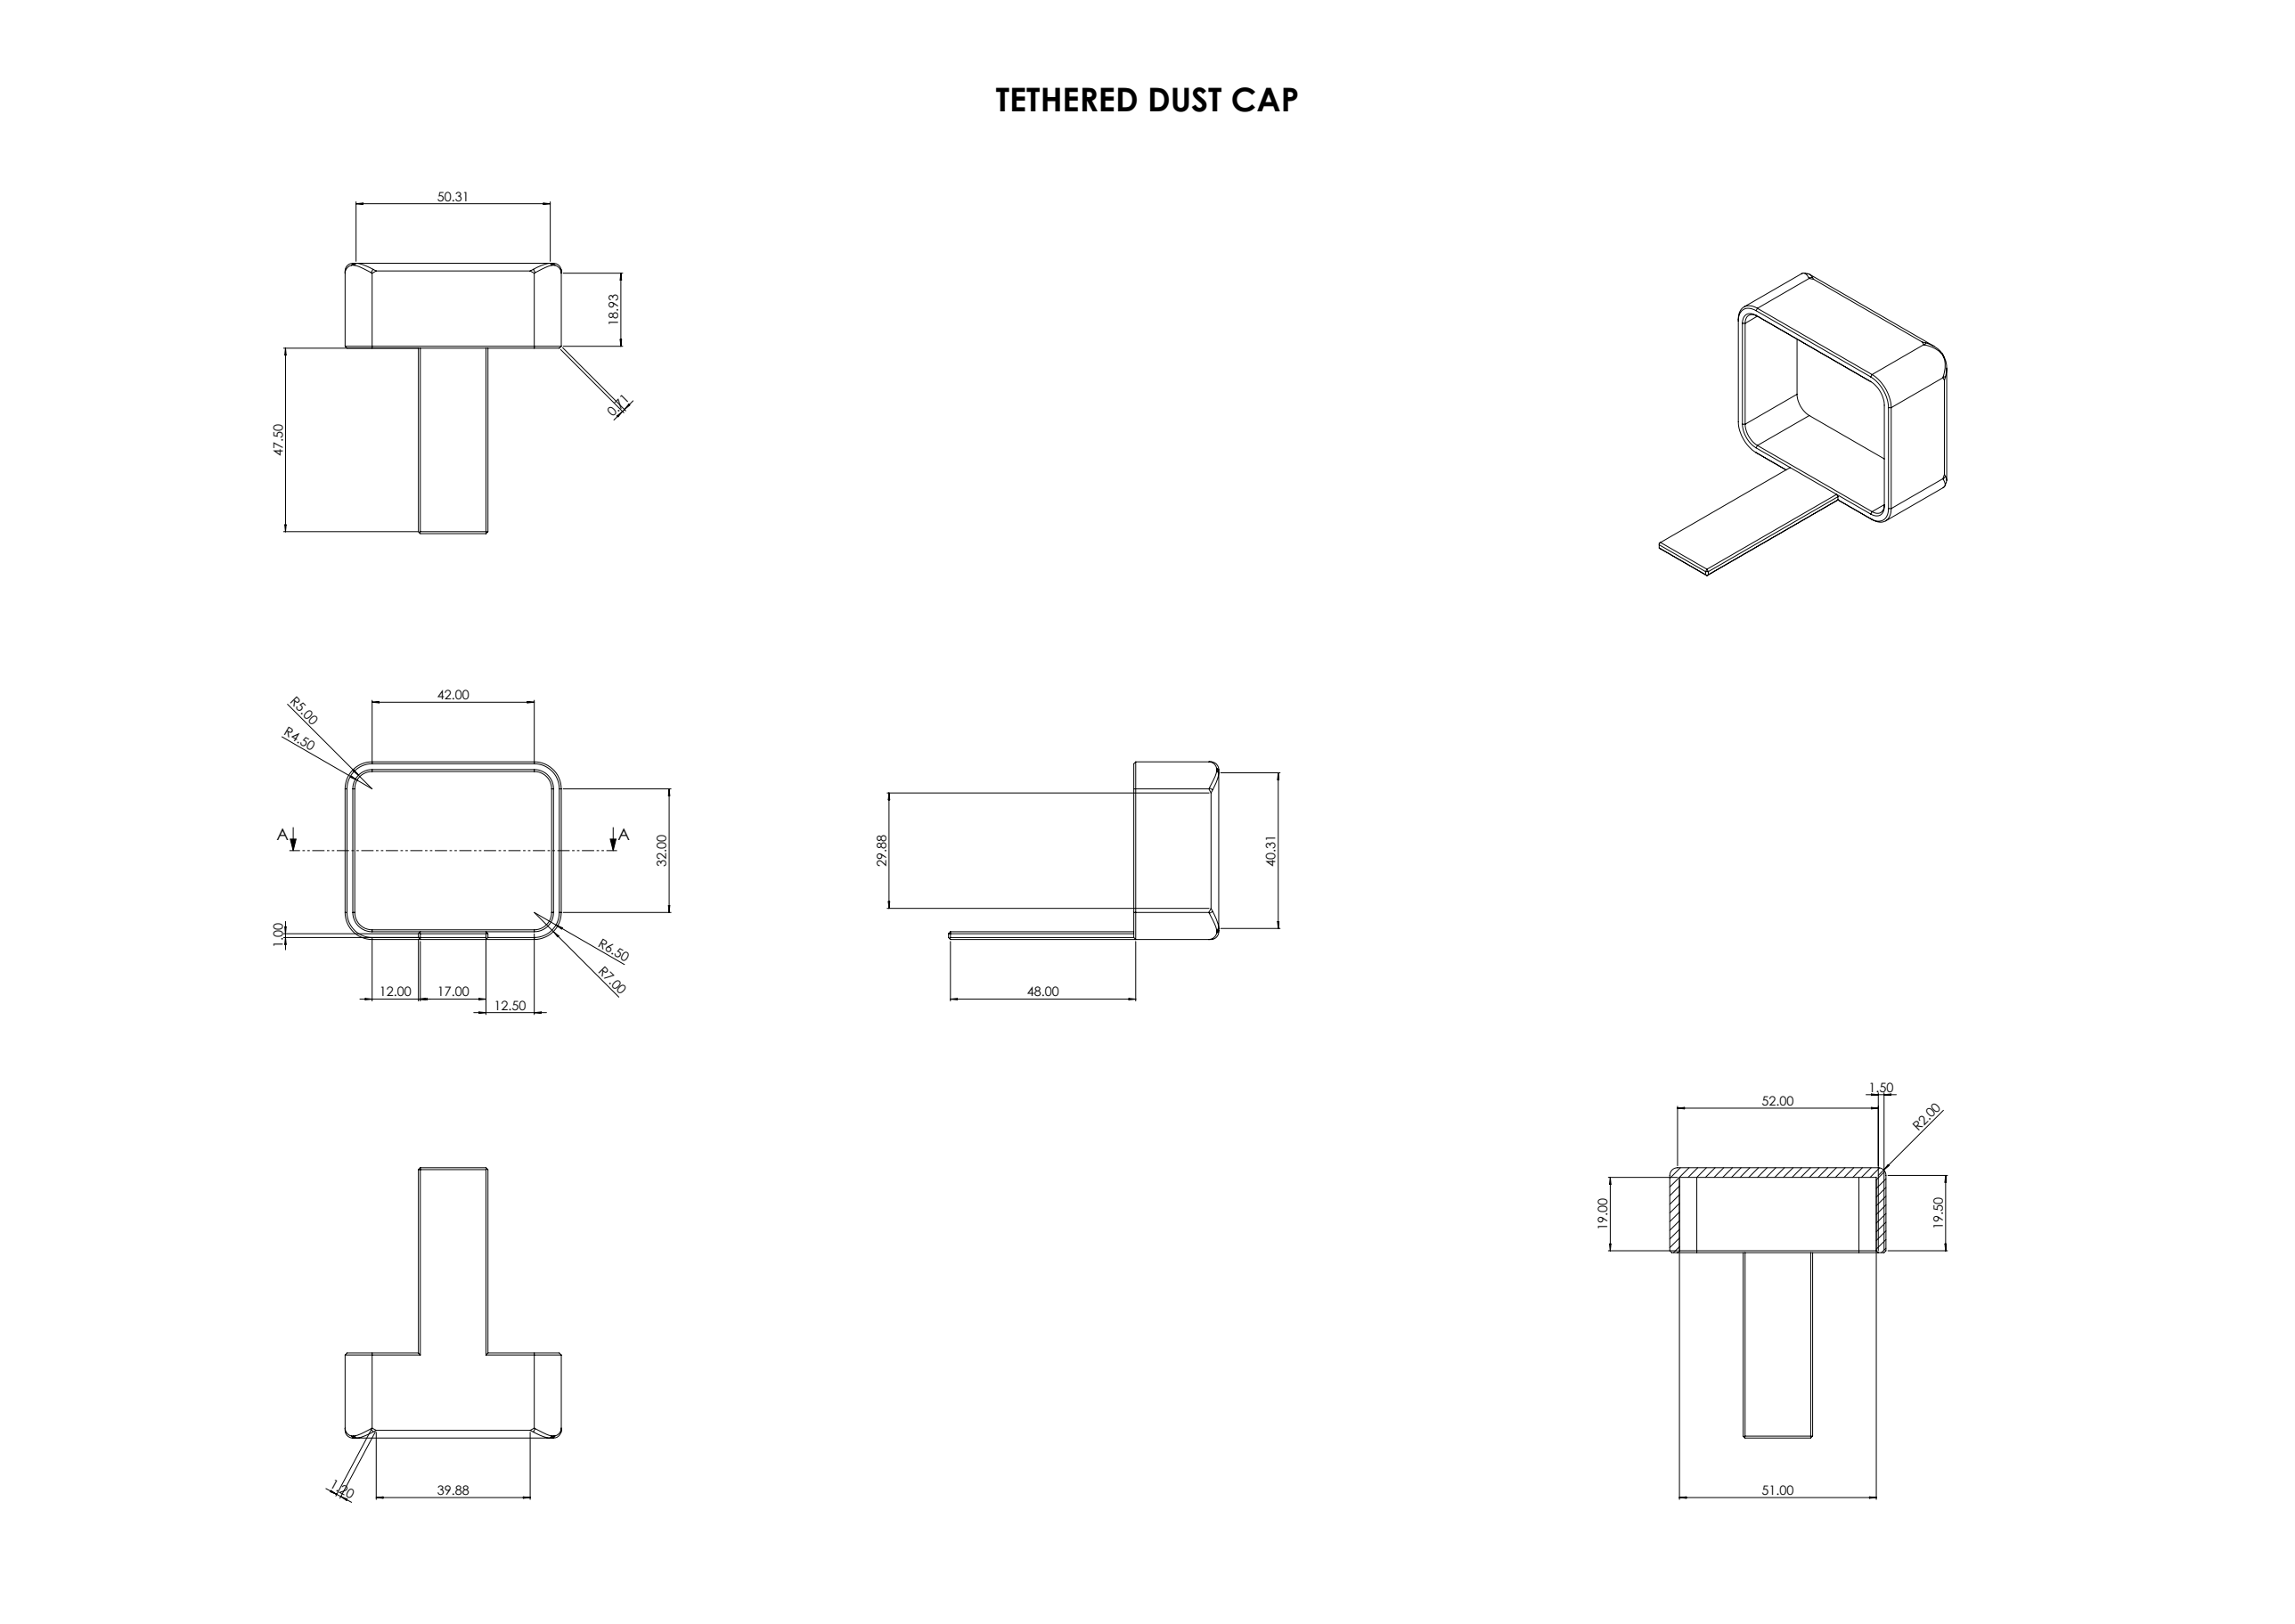
ISO-10303-21;
HEADER;
/* Generated by software containing ST-Developer
 * from STEP Tools, Inc. (www.steptools.com) 
 */

FILE_DESCRIPTION(
/* description */ (''),
/* implementation_level */ '2;1');

FILE_NAME(
/* name */ '14_Tethered_Dust_Cap.step',
/* time_stamp */ '2026-10-25T01:30:15-07:00',
/* author */ (''),
/* organization */ (''),
/* preprocessor_version */ 'ST-DEVELOPER v20.2',
/* originating_system */ 'Autodesk Translation Framework v15.15.0.0',
/* authorisation */ '');

FILE_SCHEMA (('AUTOMOTIVE_DESIGN { 1 0 10303 214 3 1 1 }'));
ENDSEC;

DATA;
#10=MECHANICAL_DESIGN_GEOMETRIC_PRESENTATION_REPRESENTATION('',(#575),#32309);
#87=(
BOUNDED_CURVE()
B_SPLINE_CURVE(3,(#30768,#30769,#30770,#30771,#30772,#30773,#30774,#30775,
#30776,#30777,#30778,#30779),.UNSPECIFIED.,.F.,.F.)
B_SPLINE_CURVE_WITH_KNOTS((4,2,2,2,2,4),(0.000100085581199306,0.11804875878528,
0.236101413685198,0.384034650166034,0.497829447458985,0.511841573844537),
 .UNSPECIFIED.)
CURVE()
GEOMETRIC_REPRESENTATION_ITEM()
RATIONAL_B_SPLINE_CURVE((1.,1.,1.,1.,1.,1.,1.,1.,1.,1.,1.,1.))
REPRESENTATION_ITEM('')
);
#352=B_SPLINE_CURVE_WITH_KNOTS('',3,(#29537,#29538,#29539,#29540,#29541,
#29542,#29543,#29544,#29545,#29546,#29547,#29548,#29549,#29550,#29551,#29552,
#29553,#29554,#29555,#29556,#29557,#29558,#29559,#29560,#29561,#29562,#29563,
#29564,#29565,#29566,#29567,#29568,#29569,#29570,#29571,#29572,#29573,#29574,
#29575,#29576,#29577,#29578,#29579,#29580,#29581,#29582,#29583,#29584,#29585,
#29586,#29587,#29588,#29589,#29590,#29591,#29592,#29593,#29594,#29595,#29596,
#29597,#29598,#29599,#29600,#29601,#29602,#29603,#29604,#29605,#29606,#29607,
#29608,#29609,#29610,#29611,#29612,#29613,#29614,#29615,#29616,#29617,#29618,
#29619,#29620,#29621,#29622,#29623,#29624,#29625,#29626,#29627,#29628,#29629,
#29630),.UNSPECIFIED.,.F.,.F.,(4,3,3,3,3,3,3,3,3,3,3,3,3,3,3,3,3,3,3,3,
3,3,3,3,3,3,3,3,3,3,3,4),(0.,0.0258707374451698,0.0523995842804884,0.0797001065242145,
0.108495122701971,0.138579548146388,0.170391094738405,0.204740918376836,
0.243564930469247,0.301738535677522,0.342786820776585,0.377562328700043,
0.409462754742929,0.439523776912731,0.468248829463879,0.497342034867759,
0.525270549115699,0.554941139795967,0.585586421921526,0.618112000252219,
0.653483627180876,0.694829905002005,0.747358415243329,0.784774064435163,
0.818382572828511,0.849773402002612,0.879622020764925,0.909716515573693,
0.937043932385008,0.963754510580494,0.989696242215803,1.),.UNSPECIFIED.);
#353=B_SPLINE_CURVE_WITH_KNOTS('',3,(#29632,#29633,#29634,#29635),
 .UNSPECIFIED.,.F.,.F.,(4,4),(-1.,0.),.UNSPECIFIED.);
#354=B_SPLINE_CURVE_WITH_KNOTS('',3,(#29637,#29638,#29639,#29640,#29641,
#29642,#29643,#29644,#29645,#29646,#29647,#29648,#29649,#29650,#29651,#29652,
#29653,#29654,#29655,#29656,#29657,#29658,#29659,#29660,#29661,#29662,#29663,
#29664,#29665,#29666,#29667,#29668,#29669,#29670,#29671,#29672,#29673,#29674,
#29675,#29676,#29677,#29678,#29679,#29680,#29681,#29682,#29683,#29684,#29685,
#29686,#29687,#29688,#29689,#29690,#29691,#29692,#29693,#29694,#29695,#29696,
#29697,#29698,#29699,#29700,#29701,#29702,#29703,#29704,#29705,#29706),
 .UNSPECIFIED.,.F.,.F.,(4,3,3,3,3,3,3,3,3,3,3,3,3,3,3,3,3,3,3,3,3,3,3,4),
(0.,0.0359057501184,0.0731782994099124,0.112196676257152,0.153588188584124,
0.19856311186321,0.251379995782812,0.322351118570897,0.369695903527712,
0.412227930465316,0.451958538122157,0.49032799292638,0.52995524039796,0.570194128050318,
0.613255077113093,0.66118815818441,0.72826108783719,0.783703920872222,0.829758018851651,
0.872318514138739,0.910997179683127,0.94830001070203,0.984014129742057,
1.),.UNSPECIFIED.);
#355=B_SPLINE_CURVE_WITH_KNOTS('',3,(#29742,#29743,#29744,#29745,#29746,
#29747,#29748,#29749,#29750,#29751,#29752,#29753,#29754,#29755,#29756,#29757,
#29758,#29759,#29760,#29761,#29762,#29763,#29764,#29765,#29766,#29767,#29768,
#29769,#29770,#29771,#29772,#29773,#29774,#29775,#29776,#29777,#29778,#29779,
#29780,#29781,#29782,#29783,#29784,#29785,#29786,#29787,#29788,#29789,#29790,
#29791,#29792,#29793,#29794,#29795,#29796,#29797,#29798,#29799,#29800,#29801,
#29802,#29803,#29804,#29805,#29806,#29807,#29808,#29809,#29810,#29811),
 .UNSPECIFIED.,.F.,.F.,(4,3,3,3,3,3,3,3,3,3,3,3,3,3,3,3,3,3,3,3,3,3,3,4),
(0.,0.0359049134463849,0.073176547549646,0.112193893168169,0.153584182812285,
0.198557501853783,0.251370838267118,0.322351741442161,0.369695708180622,
0.412227003870618,0.451956929703973,0.490325803323821,0.529954284988624,
0.570193684366073,0.613255163900098,0.661188823039329,0.728261735081395,
0.783705956052361,0.829760865743545,0.872320649307659,0.91099999721276,
0.948303461797003,0.984018202039666,1.),.UNSPECIFIED.);
#356=B_SPLINE_CURVE_WITH_KNOTS('',3,(#29813,#29814,#29815,#29816),
 .UNSPECIFIED.,.F.,.F.,(4,4),(0.,1.),.UNSPECIFIED.);
#357=B_SPLINE_CURVE_WITH_KNOTS('',3,(#29818,#29819,#29820,#29821,#29822,
#29823,#29824,#29825,#29826,#29827,#29828,#29829,#29830,#29831,#29832,#29833,
#29834,#29835,#29836,#29837,#29838,#29839,#29840,#29841,#29842,#29843,#29844,
#29845,#29846,#29847,#29848,#29849,#29850,#29851,#29852,#29853,#29854,#29855,
#29856,#29857,#29858,#29859,#29860,#29861,#29862,#29863,#29864,#29865,#29866,
#29867,#29868,#29869,#29870,#29871,#29872,#29873,#29874,#29875,#29876,#29877,
#29878,#29879,#29880,#29881,#29882,#29883,#29884,#29885,#29886,#29887,#29888,
#29889,#29890,#29891,#29892,#29893,#29894,#29895,#29896,#29897,#29898,#29899,
#29900,#29901,#29902,#29903,#29904,#29905,#29906,#29907,#29908,#29909,#29910,
#29911),.UNSPECIFIED.,.F.,.F.,(4,3,3,3,3,3,3,3,3,3,3,3,3,3,3,3,3,3,3,3,
3,3,3,3,3,3,3,3,3,3,3,4),(0.,0.0258806755131893,0.0524200922167716,0.0797320051430074,
0.108539985769749,0.138639209785132,0.170468542508365,0.204841962640731,
0.243705620941324,0.301747786726151,0.342801252332619,0.377583664170473,
0.409491204995713,0.439559328397146,0.468291405426299,0.497246492955408,
0.525185050106943,0.554860984475259,0.585493446299901,0.618003829089383,
0.653355383451557,0.694654043666211,0.747235195717053,0.784647728535492,
0.818250751836891,0.849635399921593,0.879477588119271,0.909608191089453,
0.936927404966159,0.963630037681853,0.989563296559285,1.),.UNSPECIFIED.);
#358=B_SPLINE_CURVE_WITH_KNOTS('',3,(#29934,#29935,#29936,#29937,#29938),
 .UNSPECIFIED.,.F.,.F.,(4,1,4),(0.000100085581199305,0.2925237931603,0.511841573844625),
 .UNSPECIFIED.);
#359=B_SPLINE_CURVE_WITH_KNOTS('',3,(#29941,#29942,#29943,#29944,#29945),
 .UNSPECIFIED.,.F.,.F.,(4,1,4),(-0.511841573844625,-0.2925237931603,-0.000100085581199305),
 .UNSPECIFIED.);
#360=B_SPLINE_CURVE_WITH_KNOTS('',3,(#29971,#29972,#29973,#29974),
 .UNSPECIFIED.,.F.,.F.,(4,4),(-0.568951195767079,-0.511841573844535),
 .UNSPECIFIED.);
#361=B_SPLINE_CURVE_WITH_KNOTS('',3,(#29975,#29976,#29977,#29978),
 .UNSPECIFIED.,.F.,.F.,(4,4),(0.511841573844535,0.568951195767079),
 .UNSPECIFIED.);
#362=B_SPLINE_CURVE_WITH_KNOTS('',3,(#30000,#30001,#30002,#30003,#30004),
 .UNSPECIFIED.,.F.,.F.,(4,1,4),(-1.80301165508774,-1.58369377785584,-1.29126994154665),
 .UNSPECIFIED.);
#363=B_SPLINE_CURVE_WITH_KNOTS('',3,(#30007,#30008,#30009,#30010,#30011),
 .UNSPECIFIED.,.F.,.F.,(4,1,4),(1.29126994154665,1.58369377785584,1.80301165508774),
 .UNSPECIFIED.);
#364=B_SPLINE_CURVE_WITH_KNOTS('',3,(#30028,#30029,#30030,#30031),
 .UNSPECIFIED.,.F.,.F.,(4,4),(-1.29126994154674,-1.2341603196242),
 .UNSPECIFIED.);
#365=B_SPLINE_CURVE_WITH_KNOTS('',3,(#30032,#30033,#30034,#30035),
 .UNSPECIFIED.,.F.,.F.,(4,4),(1.2341603196242,1.29126994154674),
 .UNSPECIFIED.);
#366=B_SPLINE_CURVE_WITH_KNOTS('',3,(#30040,#30041,#30042,#30043,#30044,
#30045,#30046,#30047,#30048,#30049,#30050,#30051,#30052,#30053,#30054,#30055,
#30056,#30057,#30058,#30059,#30060,#30061,#30062,#30063,#30064,#30065,#30066,
#30067,#30068,#30069,#30070,#30071,#30072,#30073,#30074,#30075,#30076,#30077,
#30078,#30079,#30080,#30081,#30082,#30083,#30084,#30085,#30086,#30087,#30088,
#30089,#30090,#30091,#30092,#30093,#30094,#30095,#30096,#30097,#30098,#30099,
#30100,#30101,#30102,#30103,#30104,#30105,#30106,#30107,#30108,#30109,#30110,
#30111,#30112,#30113,#30114,#30115,#30116,#30117,#30118,#30119,#30120,#30121,
#30122,#30123,#30124,#30125,#30126,#30127,#30128,#30129,#30130,#30131,#30132,
#30133),.UNSPECIFIED.,.F.,.F.,(4,3,3,3,3,3,3,3,3,3,3,3,3,3,3,3,3,3,3,3,
3,3,3,3,3,3,3,3,3,3,3,4),(0.,0.0258806755478976,0.0524200922876265,0.0797320052517776,
0.108539985919231,0.138639209979136,0.170468542753168,0.204841962945636,
0.243705621312987,0.301747784910779,0.34280125092102,0.377583662940723,
0.409491203889412,0.439559327385709,0.468291404493187,0.49724649358827,
0.525185050645796,0.554860984980434,0.585493446871105,0.61800382974593,
0.653355384235859,0.694654044834357,0.747235196465702,0.78464772923462,
0.818250752522057,0.849635400605874,0.879477588809083,0.909608191606812,
0.936927405502566,0.963630038237505,0.989563297137722,1.),.UNSPECIFIED.);
#367=B_SPLINE_CURVE_WITH_KNOTS('',3,(#30135,#30136,#30137,#30138,#30139),
 .UNSPECIFIED.,.F.,.F.,(4,1,4),(-0.511841573844626,-0.2925237931603,-0.000100085581199306),
 .UNSPECIFIED.);
#368=B_SPLINE_CURVE_WITH_KNOTS('',3,(#30195,#30196,#30197,#30198,#30199,
#30200,#30201,#30202,#30203,#30204,#30205,#30206,#30207,#30208,#30209,#30210,
#30211,#30212,#30213,#30214,#30215,#30216,#30217,#30218,#30219,#30220,#30221,
#30222,#30223,#30224,#30225,#30226,#30227,#30228,#30229,#30230,#30231,#30232,
#30233,#30234,#30235,#30236,#30237,#30238,#30239,#30240,#30241,#30242,#30243,
#30244,#30245,#30246,#30247,#30248,#30249,#30250,#30251,#30252,#30253,#30254,
#30255,#30256,#30257,#30258,#30259,#30260,#30261,#30262,#30263,#30264,#30265,
#30266,#30267,#30268,#30269,#30270,#30271,#30272,#30273,#30274,#30275,#30276,
#30277,#30278,#30279,#30280,#30281,#30282,#30283,#30284,#30285,#30286,#30287,
#30288),.UNSPECIFIED.,.F.,.F.,(4,3,3,3,3,3,3,3,3,3,3,3,3,3,3,3,3,3,3,3,
3,3,3,3,3,3,3,3,3,3,3,4),(0.,0.0258707373852982,0.0523995841574412,0.0797001063343714,
0.108495122436769,0.138579547796529,0.170391094289058,0.204740917798661,
0.243564929672972,0.301738533531649,0.342786818919582,0.377562326926431,
0.409462753002346,0.439523775182168,0.468248827730827,0.497342036568372,
0.525270550411946,0.554941141011199,0.585586423119629,0.618112001453677,
0.653483628442009,0.694829906775482,0.747358417163163,0.784774066048828,
0.818382574240286,0.849773403259427,0.87962202189283,0.909716516419622,
0.937043933139065,0.963754511246871,0.989696242803908,1.),.UNSPECIFIED.);
#369=B_SPLINE_CURVE_WITH_KNOTS('',3,(#30290,#30291,#30292,#30293),
 .UNSPECIFIED.,.F.,.F.,(4,4),(-1.,0.),.UNSPECIFIED.);
#370=B_SPLINE_CURVE_WITH_KNOTS('',3,(#30295,#30296,#30297,#30298,#30299,
#30300,#30301,#30302,#30303,#30304,#30305,#30306,#30307,#30308,#30309,#30310,
#30311,#30312,#30313,#30314,#30315,#30316,#30317,#30318,#30319,#30320,#30321,
#30322,#30323,#30324,#30325,#30326,#30327,#30328,#30329,#30330,#30331,#30332,
#30333,#30334,#30335,#30336,#30337,#30338,#30339,#30340,#30341,#30342,#30343,
#30344,#30345,#30346,#30347,#30348,#30349,#30350,#30351,#30352,#30353,#30354,
#30355,#30356,#30357,#30358,#30359,#30360,#30361,#30362,#30363,#30364),
 .UNSPECIFIED.,.F.,.F.,(4,3,3,3,3,3,3,3,3,3,3,3,3,3,3,3,3,3,3,3,3,3,3,4),
(0.,0.0359057503974645,0.0731782999903264,0.112196677171334,0.153588189884582,
0.198563113652405,0.251379998572626,0.322351119089413,0.369695904344816,
0.412227931549056,0.45195853945437,0.490327994460789,0.529955241857638,
0.570194129909524,0.613255079462038,0.661188161329761,0.728261095682754,
0.783703926991951,0.829758024663586,0.872318518497689,0.910997184172885,
0.948300015335705,0.984014134572557,1.),.UNSPECIFIED.);
#371=B_SPLINE_CURVE_WITH_KNOTS('',3,(#30399,#30400,#30401,#30402,#30403,
#30404,#30405,#30406,#30407,#30408,#30409,#30410,#30411,#30412,#30413,#30414,
#30415,#30416,#30417,#30418,#30419,#30420,#30421,#30422,#30423,#30424,#30425,
#30426,#30427,#30428,#30429,#30430,#30431,#30432,#30433,#30434,#30435,#30436,
#30437,#30438,#30439,#30440,#30441,#30442,#30443,#30444,#30445,#30446,#30447,
#30448,#30449,#30450,#30451,#30452,#30453,#30454,#30455,#30456,#30457,#30458,
#30459,#30460,#30461,#30462,#30463,#30464,#30465,#30466,#30467,#30468),
 .UNSPECIFIED.,.F.,.F.,(4,3,3,3,3,3,3,3,3,3,3,3,3,3,3,3,3,3,3,3,3,3,3,4),
(0.,0.0359049133077996,0.0731765472614101,0.112193892714089,0.153584182166311,
0.198557500964563,0.251370836880033,0.322351741174105,0.369695707765568,
0.412227003323922,0.451956929034388,0.490325802554425,0.529954284258119,
0.5701936834371,0.613255162727241,0.661188821470719,0.728261731182501,0.783705953011855,
0.829760862856234,0.872320647142176,0.910999994982448,0.948303459495199,
0.984018199640234,1.),.UNSPECIFIED.);
#372=B_SPLINE_CURVE_WITH_KNOTS('',3,(#30469,#30470,#30471,#30472),
 .UNSPECIFIED.,.F.,.F.,(4,4),(0.,1.),.UNSPECIFIED.);
#373=B_SPLINE_CURVE_WITH_KNOTS('',3,(#30494,#30495,#30496,#30497,#30498),
 .UNSPECIFIED.,.F.,.F.,(4,1,4),(0.000100085581199306,0.2925237931603,0.511841573844626),
 .UNSPECIFIED.);
#374=B_SPLINE_CURVE_WITH_KNOTS('',3,(#30525,#30526,#30527,#30528),
 .UNSPECIFIED.,.F.,.F.,(4,4),(-0.568951195767079,-0.511841573844535),
 .UNSPECIFIED.);
#375=B_SPLINE_CURVE_WITH_KNOTS('',3,(#30529,#30530,#30531,#30532),
 .UNSPECIFIED.,.F.,.F.,(4,4),(0.511841573844535,0.568951195767079),
 .UNSPECIFIED.);
#376=B_SPLINE_CURVE_WITH_KNOTS('',3,(#30554,#30555,#30556,#30557,#30558),
 .UNSPECIFIED.,.F.,.F.,(4,1,4),(-1.82014070277373,-1.52771686646454,-1.30839898923264),
 .UNSPECIFIED.);
#377=B_SPLINE_CURVE_WITH_KNOTS('',3,(#30561,#30562,#30563,#30564,#30565),
 .UNSPECIFIED.,.F.,.F.,(4,1,4),(1.30839898923264,1.52771686646454,1.82014070277373),
 .UNSPECIFIED.);
#378=B_SPLINE_CURVE_WITH_KNOTS('',3,(#30582,#30583,#30584,#30585),
 .UNSPECIFIED.,.F.,.F.,(4,4),(-1.30839898923273,-1.25128936731019),
 .UNSPECIFIED.);
#379=B_SPLINE_CURVE_WITH_KNOTS('',3,(#30586,#30587,#30588,#30589),
 .UNSPECIFIED.,.F.,.F.,(4,4),(1.25128936731019,1.30839898923273),
 .UNSPECIFIED.);
#380=B_SPLINE_CURVE_WITH_KNOTS('',3,(#30594,#30595,#30596,#30597),
 .UNSPECIFIED.,.F.,.F.,(4,4),(-0.568951195767077,-0.511841573844537),
 .UNSPECIFIED.);
#381=B_SPLINE_CURVE_WITH_KNOTS('',3,(#30601,#30602,#30603,#30604),
 .UNSPECIFIED.,.F.,.F.,(4,4),(-1.30839898923273,-1.25128936731019),
 .UNSPECIFIED.);
#382=B_SPLINE_CURVE_WITH_KNOTS('',3,(#30608,#30609,#30610,#30611),
 .UNSPECIFIED.,.F.,.F.,(4,4),(-0.568951195767079,-0.511841573844536),
 .UNSPECIFIED.);
#383=B_SPLINE_CURVE_WITH_KNOTS('',3,(#30615,#30616,#30617,#30618),
 .UNSPECIFIED.,.F.,.F.,(4,4),(-1.29126994154674,-1.2341603196242),
 .UNSPECIFIED.);
#384=B_SPLINE_CURVE_WITH_KNOTS('',3,(#30679,#30680,#30681,#30682,#30683,
#30684,#30685,#30686,#30687,#30688,#30689,#30690,#30691,#30692,#30693,#30694,
#30695,#30696,#30697,#30698,#30699,#30700,#30701,#30702,#30703,#30704,#30705,
#30706,#30707,#30708,#30709,#30710,#30711,#30712,#30713,#30714,#30715,#30716,
#30717,#30718,#30719,#30720,#30721,#30722,#30723,#30724,#30725,#30726,#30727,
#30728,#30729,#30730,#30731,#30732,#30733,#30734,#30735,#30736,#30737,#30738,
#30739,#30740,#30741,#30742,#30743,#30744,#30745,#30746,#30747,#30748),
 .UNSPECIFIED.,.F.,.F.,(4,3,3,3,3,3,3,3,3,3,3,3,3,3,3,3,3,3,3,3,3,3,3,4),
(0.,0.0359057503975373,0.0731782999904773,0.112196677171571,0.153588189884912,
0.198563113652762,0.251379998573341,0.322351119089333,0.36969590434482,
0.412227931549108,0.451958539454481,0.490327994460949,0.529955241857821,
0.570194129909769,0.613255079462367,0.66118816133035,0.728261095684453,
0.783703926993341,0.829758024664918,0.872318518498689,0.910997184173894,
0.948300015336798,0.98401413457368,1.),.UNSPECIFIED.);
#385=B_SPLINE_CURVE_WITH_KNOTS('',3,(#30750,#30751,#30752,#30753,#30754),
 .UNSPECIFIED.,.F.,.F.,(4,1,4),(1.30839898923264,1.52771686646453,1.82014070277373),
 .UNSPECIFIED.);
#386=B_SPLINE_CURVE_WITH_KNOTS('',3,(#30756,#30757,#30758,#30759),
 .UNSPECIFIED.,.F.,.F.,(4,4),(1.25128936731019,1.30839898923273),
 .UNSPECIFIED.);
#387=B_SPLINE_CURVE_WITH_KNOTS('',3,(#30763,#30764,#30765,#30766),
 .UNSPECIFIED.,.F.,.F.,(4,4),(0.511841573844537,0.568951195767077),
 .UNSPECIFIED.);
#388=B_SPLINE_CURVE_WITH_KNOTS('',3,(#30780,#30781,#30782,#30783,#30784,
#30785,#30786,#30787,#30788,#30789,#30790,#30791,#30792,#30793,#30794,#30795,
#30796,#30797,#30798,#30799,#30800,#30801,#30802,#30803,#30804,#30805,#30806,
#30807,#30808,#30809,#30810,#30811,#30812,#30813,#30814,#30815,#30816,#30817,
#30818,#30819,#30820,#30821,#30822,#30823,#30824,#30825,#30826,#30827,#30828,
#30829,#30830,#30831,#30832,#30833,#30834,#30835,#30836,#30837,#30838,#30839,
#30840,#30841,#30842,#30843,#30844,#30845,#30846,#30847,#30848,#30849),
 .UNSPECIFIED.,.F.,.F.,(4,3,3,3,3,3,3,3,3,3,3,3,3,3,3,3,3,3,3,3,3,3,3,4),
(0.,0.0359049130301229,0.073176546683956,0.112193891804418,0.153584180872903,
0.198557499184731,0.251370834104054,0.322351740640927,0.369695706937292,
0.412227002231532,0.451956927695583,0.490325801015499,0.529954282797085,
0.570193681578136,0.613255160380649,0.661188818329747,0.72826172337588,
0.783705946924147,0.829760857074988,0.872320642806241,0.910999990516432,
0.948303454885518,0.984018194834891,1.),.UNSPECIFIED.);
#389=B_SPLINE_CURVE_WITH_KNOTS('',3,(#30894,#30895,#30896,#30897,#30898,
#30899,#30900,#30901,#30902,#30903,#30904,#30905,#30906,#30907,#30908,#30909,
#30910,#30911,#30912,#30913,#30914,#30915,#30916,#30917,#30918,#30919,#30920,
#30921,#30922,#30923,#30924,#30925,#30926,#30927,#30928,#30929,#30930,#30931,
#30932,#30933,#30934,#30935,#30936,#30937,#30938,#30939,#30940,#30941,#30942,
#30943,#30944,#30945,#30946,#30947,#30948,#30949,#30950,#30951,#30952,#30953,
#30954,#30955,#30956,#30957,#30958,#30959,#30960,#30961,#30962,#30963,#30964,
#30965,#30966,#30967,#30968,#30969,#30970,#30971,#30972,#30973,#30974,#30975,
#30976,#30977,#30978,#30979,#30980,#30981,#30982,#30983,#30984,#30985,#30986,
#30987),.UNSPECIFIED.,.F.,.F.,(4,3,3,3,3,3,3,3,3,3,3,3,3,3,3,3,3,3,3,3,
3,3,3,3,3,3,3,3,3,3,3,4),(0.,0.0258707373554823,0.0523995840965019,0.0797001062399438,
0.108495122304716,0.13857954762218,0.170391094064582,0.204740917510112,
0.243564929276073,0.301738532460215,0.342786817991936,0.377562326039311,
0.409462752131609,0.4395237743171,0.468248826864701,0.497342037419088,0.525270551060381,
0.554941141619107,0.585586423719045,0.618112002054742,0.653483629073077,
0.694829907664093,0.747358418123701,0.784774066856292,0.818382574947157,
0.849773403889227,0.879622022458522,0.909716516843892,0.937043933517235,
0.963754511581492,0.989696243099283,1.),.UNSPECIFIED.);
#390=B_SPLINE_CURVE_WITH_KNOTS('',3,(#30989,#30990,#30991,#30992),
 .UNSPECIFIED.,.F.,.F.,(4,4),(-1.,0.),.UNSPECIFIED.);
#391=B_SPLINE_CURVE_WITH_KNOTS('',3,(#30994,#30995,#30996,#30997,#30998,
#30999,#31000,#31001,#31002,#31003,#31004,#31005,#31006,#31007,#31008,#31009,
#31010,#31011,#31012,#31013,#31014,#31015,#31016,#31017,#31018,#31019,#31020,
#31021,#31022,#31023,#31024,#31025,#31026,#31027,#31028,#31029,#31030,#31031,
#31032,#31033,#31034,#31035,#31036,#31037,#31038,#31039,#31040,#31041,#31042,
#31043,#31044,#31045,#31046,#31047,#31048,#31049,#31050,#31051,#31052,#31053,
#31054,#31055,#31056,#31057,#31058,#31059,#31060,#31061,#31062,#31063),
 .UNSPECIFIED.,.F.,.F.,(4,3,3,3,3,3,3,3,3,3,3,3,3,3,3,3,3,3,3,3,3,3,3,4),
(0.,0.0359057505369141,0.0731783002803435,0.112196677628097,0.153588190534333,
0.19856311454628,0.251379999966526,0.322351119348276,0.369695904752862,
0.412227932090299,0.451958540119749,0.490327995227232,0.529955242586758,
0.570194130838204,0.613255080635413,0.66118816290105,0.728261099602057,
0.783703930049219,0.829758027567063,0.872318520675297,0.910997186415849,
0.948300017650692,0.984014136985868,1.),.UNSPECIFIED.);
#392=B_SPLINE_CURVE_WITH_KNOTS('',3,(#31099,#31100,#31101,#31102,#31103,
#31104,#31105,#31106,#31107,#31108,#31109,#31110,#31111,#31112,#31113,#31114,
#31115,#31116,#31117,#31118,#31119,#31120,#31121,#31122,#31123,#31124,#31125,
#31126,#31127,#31128,#31129,#31130,#31131,#31132,#31133,#31134,#31135,#31136,
#31137,#31138,#31139,#31140,#31141,#31142,#31143,#31144,#31145,#31146,#31147,
#31148,#31149,#31150,#31151,#31152,#31153,#31154,#31155,#31156,#31157,#31158,
#31159,#31160,#31161,#31162,#31163,#31164,#31165,#31166,#31167,#31168),
 .UNSPECIFIED.,.F.,.F.,(4,3,3,3,3,3,3,3,3,3,3,3,3,3,3,3,3,3,3,3,3,3,3,4),
(0.,0.0359049130299729,0.0731765466835763,0.112193891804017,0.153584180872098,
0.198557499183881,0.251370834102748,0.322351740640327,0.369695706936552,
0.41222700223062,0.451956927694618,0.490325801013735,0.529954282795424,
0.570193681576247,0.613255160378796,0.661188818327897,0.728261723370456,
0.783705946920119,0.829760857071578,0.872320642803683,0.910999990513864,
0.948303454883392,0.984018194832596,1.),.UNSPECIFIED.);
#393=B_SPLINE_CURVE_WITH_KNOTS('',3,(#31170,#31171,#31172,#31173),
 .UNSPECIFIED.,.F.,.F.,(4,4),(0.,1.),.UNSPECIFIED.);
#394=B_SPLINE_CURVE_WITH_KNOTS('',3,(#31175,#31176,#31177,#31178,#31179,
#31180,#31181,#31182,#31183,#31184,#31185,#31186,#31187,#31188,#31189,#31190,
#31191,#31192,#31193,#31194,#31195,#31196,#31197,#31198,#31199,#31200,#31201,
#31202,#31203,#31204,#31205,#31206,#31207,#31208,#31209,#31210,#31211,#31212,
#31213,#31214,#31215,#31216,#31217,#31218,#31219,#31220,#31221,#31222,#31223,
#31224,#31225,#31226,#31227,#31228,#31229,#31230,#31231,#31232,#31233,#31234,
#31235,#31236,#31237,#31238,#31239,#31240,#31241,#31242,#31243,#31244,#31245,
#31246,#31247,#31248,#31249,#31250,#31251,#31252,#31253,#31254,#31255,#31256,
#31257,#31258,#31259,#31260,#31261,#31262,#31263,#31264,#31265,#31266,#31267,
#31268),.UNSPECIFIED.,.F.,.F.,(4,3,3,3,3,3,3,3,3,3,3,3,3,3,3,3,3,3,3,3,
3,3,3,3,3,3,3,3,3,3,3,4),(0.,0.0258806756174258,0.052420092429605,0.0797320054697036,
0.108539986218788,0.138639210368191,0.170468543243868,0.204841963556246,
0.243705622058159,0.301747781272309,0.342801248093589,0.377583660478043,
0.409491201673175,0.439559325359787,0.468291402624354,0.497246494854993,
0.525185051724753,0.554860985991956,0.585493448014801,0.618003831060507,
0.653355385806342,0.694654047173711,0.747235197965173,0.78464773063489,
0.818250753894271,0.849635401976391,0.879477590190491,0.909608192642869,
0.936927406576889,0.963630039350146,0.989563298296144,1.),.UNSPECIFIED.);
#395=B_SPLINE_CURVE_WITH_KNOTS('',3,(#31291,#31292,#31293,#31294,#31295),
 .UNSPECIFIED.,.F.,.F.,(4,1,4),(0.000100085581199305,0.2925237931603,0.511841573844626),
 .UNSPECIFIED.);
#396=B_SPLINE_CURVE_WITH_KNOTS('',3,(#31297,#31298,#31299,#31300,#31301),
 .UNSPECIFIED.,.F.,.F.,(4,1,4),(-0.511841573844626,-0.2925237931603,-0.000100085581199305),
 .UNSPECIFIED.);
#397=B_SPLINE_CURVE_WITH_KNOTS('',3,(#31324,#31325,#31326,#31327),
 .UNSPECIFIED.,.F.,.F.,(4,4),(0.511841573844536,0.568951195767079),
 .UNSPECIFIED.);
#398=B_SPLINE_CURVE_WITH_KNOTS('',3,(#31348,#31349,#31350,#31351,#31352),
 .UNSPECIFIED.,.F.,.F.,(4,1,4),(-1.80301165508774,-1.58369377785584,-1.29126994154665),
 .UNSPECIFIED.);
#399=B_SPLINE_CURVE_WITH_KNOTS('',3,(#31355,#31356,#31357,#31358,#31359),
 .UNSPECIFIED.,.F.,.F.,(4,1,4),(1.29126994154665,1.58369377785584,1.80301165508774),
 .UNSPECIFIED.);
#400=B_SPLINE_CURVE_WITH_KNOTS('',3,(#31376,#31377,#31378,#31379),
 .UNSPECIFIED.,.F.,.F.,(4,4),(1.2341603196242,1.29126994154674),
 .UNSPECIFIED.);
#401=B_SPLINE_CURVE_WITH_KNOTS('',3,(#31428,#31429,#31430,#31431,#31432,
#31433,#31434,#31435,#31436,#31437,#31438,#31439,#31440,#31441,#31442,#31443,
#31444,#31445,#31446,#31447,#31448,#31449,#31450,#31451,#31452,#31453,#31454,
#31455,#31456,#31457,#31458,#31459,#31460,#31461,#31462,#31463,#31464,#31465,
#31466,#31467,#31468,#31469,#31470,#31471,#31472,#31473,#31474,#31475,#31476,
#31477,#31478,#31479,#31480,#31481,#31482,#31483,#31484,#31485,#31486,#31487,
#31488,#31489,#31490,#31491,#31492,#31493,#31494,#31495,#31496,#31497,#31498,
#31499,#31500,#31501,#31502,#31503,#31504,#31505,#31506,#31507,#31508,#31509,
#31510,#31511,#31512,#31513,#31514,#31515,#31516,#31517,#31518,#31519,#31520,
#31521),.UNSPECIFIED.,.F.,.F.,(4,3,3,3,3,3,3,3,3,3,3,3,3,3,3,3,3,3,3,3,
3,3,3,3,3,3,3,3,3,3,3,4),(0.,0.0258707373851967,0.0523995841581851,0.0797001063345152,
0.108495122436992,0.138579547796862,0.17039109428924,0.204740917798925,
0.243564929673233,0.301738533531212,0.342786818919031,0.377562326926076,
0.409462753001591,0.439523775181584,0.468248827730322,0.497342036568899,
0.525270550411958,0.554941141011211,0.585586423119647,0.618112001453771,
0.653483628441857,0.694829906775598,0.747358417163864,0.784774066049438,
0.818382574241438,0.849773403260588,0.879622021894085,0.909716516420564,
0.937043933139874,0.963754511247475,0.98969624280447,1.),.UNSPECIFIED.);
#402=B_SPLINE_CURVE_WITH_KNOTS('',3,(#31522,#31523,#31524,#31525),
 .UNSPECIFIED.,.F.,.F.,(4,4),(-1.,0.),.UNSPECIFIED.);
#403=B_SPLINE_CURVE_WITH_KNOTS('',3,(#31560,#31561,#31562,#31563),
 .UNSPECIFIED.,.F.,.F.,(4,4),(0.,1.),.UNSPECIFIED.);
#404=B_SPLINE_CURVE_WITH_KNOTS('',3,(#31564,#31565,#31566,#31567,#31568,
#31569,#31570,#31571,#31572,#31573,#31574,#31575,#31576,#31577,#31578,#31579,
#31580,#31581,#31582,#31583,#31584,#31585,#31586,#31587,#31588,#31589,#31590,
#31591,#31592,#31593,#31594,#31595,#31596,#31597,#31598,#31599,#31600,#31601,
#31602,#31603,#31604,#31605,#31606,#31607,#31608,#31609,#31610,#31611,#31612,
#31613,#31614,#31615,#31616,#31617,#31618,#31619,#31620,#31621,#31622,#31623,
#31624,#31625,#31626,#31627,#31628,#31629,#31630,#31631,#31632,#31633,#31634,
#31635,#31636,#31637,#31638,#31639,#31640,#31641,#31642,#31643,#31644,#31645,
#31646,#31647,#31648,#31649,#31650,#31651,#31652,#31653,#31654,#31655,#31656,
#31657),.UNSPECIFIED.,.F.,.F.,(4,3,3,3,3,3,3,3,3,3,3,3,3,3,3,3,3,3,3,3,
3,3,3,3,3,3,3,3,3,3,3,4),(0.,0.0258806756174331,0.0524200924297352,0.0797320054696585,
0.108539986218731,0.13863921036807,0.170468543243706,0.204841963556146,
0.243705622058077,0.301747781273792,0.342801248094138,0.377583660478468,
0.409491201673628,0.439559325360195,0.468291402624606,0.497246494854655,
0.52518505172447,0.554860985991691,0.585493448014516,0.61800383106021,0.653355385806122,
0.694654047173536,0.747235197964895,0.784647730634614,0.818250753893958,
0.849635401976054,0.879477590190265,0.909608192642699,0.936927406576695,
0.963630039349939,0.989563298295856,1.),.UNSPECIFIED.);
#405=B_SPLINE_CURVE_WITH_KNOTS('',3,(#31679,#31680,#31681,#31682,#31683),
 .UNSPECIFIED.,.F.,.F.,(4,1,4),(-0.511841573844627,-0.292523793160301,-0.000100085581199306),
 .UNSPECIFIED.);
#406=B_SPLINE_CURVE_WITH_KNOTS('',3,(#31723,#31724,#31725,#31726,#31727),
 .UNSPECIFIED.,.F.,.F.,(4,1,4),(-1.82014070277373,-1.52771686646453,-1.30839898923264),
 .UNSPECIFIED.);
#511=B_SPLINE_SURFACE_WITH_KNOTS('',3,3,((#29503,#29504,#29505,#29506,#29507,
#29508,#29509,#29510),(#29511,#29512,#29513,#29514,#29515,#29516,#29517,
#29518),(#29519,#29520,#29521,#29522,#29523,#29524,#29525,#29526),(#29527,
#29528,#29529,#29530,#29531,#29532,#29533,#29534)),.UNSPECIFIED.,.F.,.F.,
 .F.,(4,4),(4,1,1,1,1,4),(0.,1.),(0.,0.142857142857143,0.428571428571429,
0.571428571428571,0.857142857142857,1.),.UNSPECIFIED.);
#512=B_SPLINE_SURFACE_WITH_KNOTS('',3,3,((#29708,#29709,#29710,#29711,#29712,
#29713,#29714,#29715),(#29716,#29717,#29718,#29719,#29720,#29721,#29722,
#29723),(#29724,#29725,#29726,#29727,#29728,#29729,#29730,#29731),(#29732,
#29733,#29734,#29735,#29736,#29737,#29738,#29739)),.UNSPECIFIED.,.F.,.F.,
 .F.,(4,4),(4,1,1,1,1,4),(0.,1.),(0.,0.142857142857143,0.428571428571429,
0.571428571428571,0.857142857142857,1.),.UNSPECIFIED.);
#513=B_SPLINE_SURFACE_WITH_KNOTS('',3,3,((#29913,#29914,#29915,#29916,#29917),
(#29918,#29919,#29920,#29921,#29922),(#29923,#29924,#29925,#29926,#29927),
(#29928,#29929,#29930,#29931,#29932)),.UNSPECIFIED.,.F.,.F.,.F.,(4,4),(4,
1,4),(0.,1.),(0.000100085581199305,0.2925237931603,0.511841573844625),
 .UNSPECIFIED.);
#514=B_SPLINE_SURFACE_WITH_KNOTS('',3,3,((#29955,#29956,#29957,#29958),
(#29959,#29960,#29961,#29962),(#29963,#29964,#29965,#29966),(#29967,#29968,
#29969,#29970)),.UNSPECIFIED.,.F.,.F.,.F.,(4,4),(4,4),(0.,1.),(0.511841573844535,
0.568951195767079),.UNSPECIFIED.);
#515=B_SPLINE_SURFACE_WITH_KNOTS('',3,3,((#29979,#29980,#29981,#29982,#29983),
(#29984,#29985,#29986,#29987,#29988),(#29989,#29990,#29991,#29992,#29993),
(#29994,#29995,#29996,#29997,#29998)),.UNSPECIFIED.,.F.,.F.,.F.,(4,4),(4,
1,4),(0.,1.),(1.29126994154665,1.58369377785584,1.80301165508774),
 .UNSPECIFIED.);
#516=B_SPLINE_SURFACE_WITH_KNOTS('',3,3,((#30012,#30013,#30014,#30015),
(#30016,#30017,#30018,#30019),(#30020,#30021,#30022,#30023),(#30024,#30025,
#30026,#30027)),.UNSPECIFIED.,.F.,.F.,.F.,(4,4),(4,4),(0.,1.),(1.2341603196242,
1.29126994154674),.UNSPECIFIED.);
#517=B_SPLINE_SURFACE_WITH_KNOTS('',3,3,((#30153,#30154,#30155,#30156,#30157,
#30158,#30159,#30160,#30161,#30162),(#30163,#30164,#30165,#30166,#30167,
#30168,#30169,#30170,#30171,#30172),(#30173,#30174,#30175,#30176,#30177,
#30178,#30179,#30180,#30181,#30182),(#30183,#30184,#30185,#30186,#30187,
#30188,#30189,#30190,#30191,#30192)),.UNSPECIFIED.,.F.,.F.,.F.,(4,4),(4,
1,1,1,1,1,1,4),(0.,1.),(0.,0.0714285714285714,0.142857142857143,0.428571428571429,
0.571428571428571,0.857142857142857,0.928571428571429,1.),.UNSPECIFIED.);
#518=B_SPLINE_SURFACE_WITH_KNOTS('',3,3,((#30366,#30367,#30368,#30369,#30370,
#30371,#30372,#30373),(#30374,#30375,#30376,#30377,#30378,#30379,#30380,
#30381),(#30382,#30383,#30384,#30385,#30386,#30387,#30388,#30389),(#30390,
#30391,#30392,#30393,#30394,#30395,#30396,#30397)),.UNSPECIFIED.,.F.,.F.,
 .F.,(4,4),(4,1,1,1,1,4),(0.,1.),(0.,0.142857142857143,0.428571428571429,
0.571428571428571,0.857142857142857,1.),.UNSPECIFIED.);
#519=B_SPLINE_SURFACE_WITH_KNOTS('',3,3,((#30473,#30474,#30475,#30476,#30477),
(#30478,#30479,#30480,#30481,#30482),(#30483,#30484,#30485,#30486,#30487),
(#30488,#30489,#30490,#30491,#30492)),.UNSPECIFIED.,.F.,.F.,.F.,(4,4),(4,
1,4),(0.,1.),(0.000100085581199306,0.2925237931603,0.511841573844626),
 .UNSPECIFIED.);
#520=B_SPLINE_SURFACE_WITH_KNOTS('',3,3,((#30509,#30510,#30511,#30512),
(#30513,#30514,#30515,#30516),(#30517,#30518,#30519,#30520),(#30521,#30522,
#30523,#30524)),.UNSPECIFIED.,.F.,.F.,.F.,(4,4),(4,4),(0.,1.),(0.511841573844535,
0.568951195767079),.UNSPECIFIED.);
#521=B_SPLINE_SURFACE_WITH_KNOTS('',3,3,((#30533,#30534,#30535,#30536,#30537),
(#30538,#30539,#30540,#30541,#30542),(#30543,#30544,#30545,#30546,#30547),
(#30548,#30549,#30550,#30551,#30552)),.UNSPECIFIED.,.F.,.F.,.F.,(4,4),(4,
1,4),(0.,1.),(1.30839898923264,1.52771686646454,1.82014070277373),
 .UNSPECIFIED.);
#522=B_SPLINE_SURFACE_WITH_KNOTS('',3,3,((#30566,#30567,#30568,#30569),
(#30570,#30571,#30572,#30573),(#30574,#30575,#30576,#30577),(#30578,#30579,
#30580,#30581)),.UNSPECIFIED.,.F.,.F.,.F.,(4,4),(4,4),(0.,1.),(1.25128936731019,
1.30839898923273),.UNSPECIFIED.);
#523=B_SPLINE_SURFACE_WITH_KNOTS('',3,3,((#30852,#30853,#30854,#30855,#30856,
#30857,#30858,#30859,#30860,#30861),(#30862,#30863,#30864,#30865,#30866,
#30867,#30868,#30869,#30870,#30871),(#30872,#30873,#30874,#30875,#30876,
#30877,#30878,#30879,#30880,#30881),(#30882,#30883,#30884,#30885,#30886,
#30887,#30888,#30889,#30890,#30891)),.UNSPECIFIED.,.F.,.F.,.F.,(4,4),(4,
1,1,1,1,1,1,4),(0.,1.),(0.,0.0714285714285714,0.142857142857143,0.428571428571429,
0.571428571428571,0.857142857142857,0.928571428571429,1.),.UNSPECIFIED.);
#524=B_SPLINE_SURFACE_WITH_KNOTS('',3,3,((#31065,#31066,#31067,#31068,#31069,
#31070,#31071,#31072),(#31073,#31074,#31075,#31076,#31077,#31078,#31079,
#31080),(#31081,#31082,#31083,#31084,#31085,#31086,#31087,#31088),(#31089,
#31090,#31091,#31092,#31093,#31094,#31095,#31096)),.UNSPECIFIED.,.F.,.F.,
 .F.,(4,4),(4,1,1,1,1,4),(0.,1.),(0.,0.142857142857143,0.428571428571429,
0.571428571428571,0.857142857142857,1.),.UNSPECIFIED.);
#525=B_SPLINE_SURFACE_WITH_KNOTS('',3,3,((#31270,#31271,#31272,#31273,#31274),
(#31275,#31276,#31277,#31278,#31279),(#31280,#31281,#31282,#31283,#31284),
(#31285,#31286,#31287,#31288,#31289)),.UNSPECIFIED.,.F.,.F.,.F.,(4,4),(4,
1,4),(0.,1.),(0.000100085581199305,0.2925237931603,0.511841573844626),
 .UNSPECIFIED.);
#526=B_SPLINE_SURFACE_WITH_KNOTS('',3,3,((#31308,#31309,#31310,#31311),
(#31312,#31313,#31314,#31315),(#31316,#31317,#31318,#31319),(#31320,#31321,
#31322,#31323)),.UNSPECIFIED.,.F.,.F.,.F.,(4,4),(4,4),(0.,1.),(0.511841573844536,
0.568951195767079),.UNSPECIFIED.);
#527=B_SPLINE_SURFACE_WITH_KNOTS('',3,3,((#31328,#31329,#31330,#31331,#31332),
(#31333,#31334,#31335,#31336,#31337),(#31338,#31339,#31340,#31341,#31342),
(#31343,#31344,#31345,#31346,#31347)),.UNSPECIFIED.,.F.,.F.,.F.,(4,4),(4,
1,4),(0.,1.),(1.29126994154665,1.58369377785584,1.80301165508774),
 .UNSPECIFIED.);
#528=B_SPLINE_SURFACE_WITH_KNOTS('',3,3,((#31360,#31361,#31362,#31363),
(#31364,#31365,#31366,#31367),(#31368,#31369,#31370,#31371),(#31372,#31373,
#31374,#31375)),.UNSPECIFIED.,.F.,.F.,.F.,(4,4),(4,4),(0.,1.),(1.2341603196242,
1.29126994154674),.UNSPECIFIED.);
#529=B_SPLINE_SURFACE_WITH_KNOTS('',3,3,((#31386,#31387,#31388,#31389,#31390,
#31391,#31392,#31393,#31394,#31395),(#31396,#31397,#31398,#31399,#31400,
#31401,#31402,#31403,#31404,#31405),(#31406,#31407,#31408,#31409,#31410,
#31411,#31412,#31413,#31414,#31415),(#31416,#31417,#31418,#31419,#31420,
#31421,#31422,#31423,#31424,#31425)),.UNSPECIFIED.,.F.,.F.,.F.,(4,4),(4,
1,1,1,1,1,1,4),(0.,1.),(0.,0.0714285714285714,0.142857142857143,0.428571428571429,
0.571428571428571,0.857142857142857,0.928571428571429,1.),.UNSPECIFIED.);
#530=B_SPLINE_SURFACE_WITH_KNOTS('',3,3,((#31527,#31528,#31529,#31530,#31531,
#31532,#31533,#31534),(#31535,#31536,#31537,#31538,#31539,#31540,#31541,
#31542),(#31543,#31544,#31545,#31546,#31547,#31548,#31549,#31550),(#31551,
#31552,#31553,#31554,#31555,#31556,#31557,#31558)),.UNSPECIFIED.,.F.,.F.,
 .F.,(4,4),(4,1,1,1,1,4),(0.,1.),(0.,0.142857142857143,0.428571428571429,
0.571428571428571,0.857142857142857,1.),.UNSPECIFIED.);
#531=B_SPLINE_SURFACE_WITH_KNOTS('',3,3,((#31658,#31659,#31660,#31661,#31662),
(#31663,#31664,#31665,#31666,#31667),(#31668,#31669,#31670,#31671,#31672),
(#31673,#31674,#31675,#31676,#31677)),.UNSPECIFIED.,.F.,.F.,.F.,(4,4),(4,
1,4),(0.,1.),(0.000100085581199306,0.292523793160301,0.511841573844627),
 .UNSPECIFIED.);
#532=B_SPLINE_SURFACE_WITH_KNOTS('',3,3,((#31687,#31688,#31689,#31690),
(#31691,#31692,#31693,#31694),(#31695,#31696,#31697,#31698),(#31699,#31700,
#31701,#31702)),.UNSPECIFIED.,.F.,.F.,.F.,(4,4),(4,4),(0.,1.),(0.511841573844537,
0.568951195767077),.UNSPECIFIED.);
#533=B_SPLINE_SURFACE_WITH_KNOTS('',3,3,((#31703,#31704,#31705,#31706,#31707),
(#31708,#31709,#31710,#31711,#31712),(#31713,#31714,#31715,#31716,#31717),
(#31718,#31719,#31720,#31721,#31722)),.UNSPECIFIED.,.F.,.F.,.F.,(4,4),(4,
1,4),(0.,1.),(1.30839898923264,1.52771686646453,1.82014070277373),
 .UNSPECIFIED.);
#534=B_SPLINE_SURFACE_WITH_KNOTS('',3,3,((#31729,#31730,#31731,#31732),
(#31733,#31734,#31735,#31736),(#31737,#31738,#31739,#31740),(#31741,#31742,
#31743,#31744)),.UNSPECIFIED.,.F.,.F.,.F.,(4,4),(4,4),(0.,1.),(1.25128936731019,
1.30839898923273),.UNSPECIFIED.);
#547=SHAPE_REPRESENTATION_RELATIONSHIP('SRR','None',#32374,#561);
#561=ADVANCED_BREP_SHAPE_REPRESENTATION('',(#589),#32307);
#575=STYLED_ITEM('',(#32495),#589);
#589=MANIFOLD_SOLID_BREP('Body1',#13816);
#760=CYLINDRICAL_SURFACE('',#14824,4.50000000000001);
#761=CYLINDRICAL_SURFACE('',#14827,4.5);
#762=CYLINDRICAL_SURFACE('',#14841,2.);
#763=CYLINDRICAL_SURFACE('',#14843,7.00000000000001);
#764=CYLINDRICAL_SURFACE('',#14867,7.00000000000001);
#765=CYLINDRICAL_SURFACE('',#14869,7.00000000000001);
#766=CYLINDRICAL_SURFACE('',#14875,2.);
#767=CYLINDRICAL_SURFACE('',#14877,7.00000000000001);
#768=CYLINDRICAL_SURFACE('',#14879,2.);
#769=CYLINDRICAL_SURFACE('',#14880,2.);
#770=CYLINDRICAL_SURFACE('',#14882,4.50000000000001);
#771=CYLINDRICAL_SURFACE('',#14885,4.50000000000002);
#1065=CIRCLE('',#14805,5.);
#1066=CIRCLE('',#14806,4.5);
#1067=CIRCLE('',#14809,5.00000000000001);
#1068=CIRCLE('',#14810,4.50000000000001);
#1069=CIRCLE('',#14813,5.00000000000002);
#1070=CIRCLE('',#14814,4.50000000000002);
#1071=CIRCLE('',#14817,5.00000000000001);
#1072=CIRCLE('',#14818,4.50000000000001);
#1073=CIRCLE('',#14820,6.50000000000001);
#1074=CIRCLE('',#14821,6.50000000000001);
#1075=CIRCLE('',#14822,6.50000000000001);
#1076=CIRCLE('',#14823,6.50000000000001);
#1077=CIRCLE('',#14825,4.50000000000001);
#1078=CIRCLE('',#14828,4.5);
#1079=CIRCLE('',#14839,7.00000000000001);
#1080=CIRCLE('',#14840,6.50000000000001);
#1081=CIRCLE('',#14844,7.00000000000001);
#1082=CIRCLE('',#14846,7.00000000000001);
#1083=CIRCLE('',#14847,6.50000000000001);
#1084=CIRCLE('',#14849,6.50000000000001);
#1085=CIRCLE('',#14850,6.50000000000001);
#1086=CIRCLE('',#14855,7.00000000000001);
#1087=CIRCLE('',#14858,7.00000000000001);
#1088=CIRCLE('',#14863,7.00000000000001);
#1089=CIRCLE('',#14870,7.00000000000001);
#1090=CIRCLE('',#14874,7.00000000000001);
#1091=CIRCLE('',#14883,4.50000000000001);
#1092=CIRCLE('',#14886,4.50000000000002);
#1228=CONICAL_SURFACE('',#14804,4.75,0.785398163397449);
#1229=CONICAL_SURFACE('',#14808,4.75000000000001,0.785398163397451);
#1230=CONICAL_SURFACE('',#14812,4.75000000000002,0.785398163397449);
#1231=CONICAL_SURFACE('',#14816,4.75000000000001,0.785398163397449);
#1232=CONICAL_SURFACE('',#14838,6.75000000000001,0.785398163397441);
#1233=CONICAL_SURFACE('',#14845,6.75000000000001,0.785398163397444);
#1234=CONICAL_SURFACE('',#14854,6.75000000000001,0.785398163397449);
#1235=CONICAL_SURFACE('',#14857,6.75000000000001,0.785398163397449);
#1236=CONICAL_SURFACE('',#14860,6.75000000000001,0.785398163397449);
#1237=CONICAL_SURFACE('',#14862,6.75000000000001,0.785398163397449);
#1238=CONICAL_SURFACE('',#14873,6.75000000000001,0.785398163397441);
#1239=CONICAL_SURFACE('',#14878,6.75000000000001,0.785398163397441);
#1866=FACE_OUTER_BOUND('',#2719,.T.);
#1867=FACE_OUTER_BOUND('',#2720,.T.);
#1868=FACE_OUTER_BOUND('',#2721,.T.);
#1869=FACE_OUTER_BOUND('',#2722,.T.);
#1870=FACE_OUTER_BOUND('',#2723,.T.);
#1871=FACE_OUTER_BOUND('',#2724,.T.);
#1872=FACE_OUTER_BOUND('',#2725,.T.);
#1873=FACE_OUTER_BOUND('',#2726,.T.);
#1874=FACE_OUTER_BOUND('',#2727,.T.);
#1875=FACE_OUTER_BOUND('',#2728,.T.);
#1876=FACE_OUTER_BOUND('',#2729,.T.);
#1877=FACE_OUTER_BOUND('',#2730,.T.);
#1878=FACE_OUTER_BOUND('',#2731,.T.);
#1879=FACE_OUTER_BOUND('',#2732,.T.);
#1880=FACE_OUTER_BOUND('',#2733,.T.);
#1881=FACE_OUTER_BOUND('',#2734,.T.);
#1882=FACE_OUTER_BOUND('',#2735,.T.);
#1883=FACE_OUTER_BOUND('',#2736,.T.);
#1884=FACE_OUTER_BOUND('',#2737,.T.);
#1885=FACE_OUTER_BOUND('',#2738,.T.);
#1886=FACE_OUTER_BOUND('',#2739,.T.);
#1887=FACE_OUTER_BOUND('',#2740,.T.);
#1888=FACE_OUTER_BOUND('',#2741,.T.);
#1889=FACE_OUTER_BOUND('',#2742,.T.);
#1890=FACE_OUTER_BOUND('',#2743,.T.);
#1891=FACE_OUTER_BOUND('',#2744,.T.);
#1892=FACE_OUTER_BOUND('',#2745,.T.);
#1893=FACE_OUTER_BOUND('',#2746,.T.);
#1894=FACE_OUTER_BOUND('',#2747,.T.);
#1895=FACE_OUTER_BOUND('',#2748,.T.);
#1896=FACE_OUTER_BOUND('',#2749,.T.);
#1897=FACE_OUTER_BOUND('',#2750,.T.);
#1898=FACE_OUTER_BOUND('',#2751,.T.);
#1899=FACE_OUTER_BOUND('',#2752,.T.);
#1900=FACE_OUTER_BOUND('',#2753,.T.);
#1901=FACE_OUTER_BOUND('',#2754,.T.);
#1902=FACE_OUTER_BOUND('',#2755,.T.);
#1903=FACE_OUTER_BOUND('',#2756,.T.);
#1904=FACE_OUTER_BOUND('',#2757,.T.);
#1905=FACE_OUTER_BOUND('',#2758,.T.);
#1906=FACE_OUTER_BOUND('',#2759,.T.);
#1907=FACE_OUTER_BOUND('',#2760,.T.);
#1908=FACE_OUTER_BOUND('',#2761,.T.);
#1909=FACE_OUTER_BOUND('',#2762,.T.);
#1910=FACE_OUTER_BOUND('',#2763,.T.);
#1911=FACE_OUTER_BOUND('',#2764,.T.);
#1912=FACE_OUTER_BOUND('',#2765,.T.);
#1913=FACE_OUTER_BOUND('',#2766,.T.);
#1914=FACE_OUTER_BOUND('',#2767,.T.);
#1915=FACE_OUTER_BOUND('',#2768,.T.);
#1916=FACE_OUTER_BOUND('',#2769,.T.);
#1917=FACE_OUTER_BOUND('',#2770,.T.);
#1918=FACE_OUTER_BOUND('',#2771,.T.);
#1919=FACE_OUTER_BOUND('',#2772,.T.);
#1920=FACE_OUTER_BOUND('',#2773,.T.);
#1921=FACE_OUTER_BOUND('',#2774,.T.);
#1922=FACE_OUTER_BOUND('',#2775,.T.);
#1923=FACE_OUTER_BOUND('',#2776,.T.);
#1924=FACE_OUTER_BOUND('',#2777,.T.);
#1925=FACE_OUTER_BOUND('',#2778,.T.);
#1926=FACE_OUTER_BOUND('',#2779,.T.);
#1927=FACE_OUTER_BOUND('',#2780,.T.);
#1928=FACE_OUTER_BOUND('',#2781,.T.);
#1929=FACE_OUTER_BOUND('',#2782,.T.);
#1930=FACE_OUTER_BOUND('',#2783,.T.);
#1931=FACE_OUTER_BOUND('',#2784,.T.);
#1932=FACE_OUTER_BOUND('',#2785,.T.);
#1933=FACE_OUTER_BOUND('',#2786,.T.);
#1934=FACE_OUTER_BOUND('',#2787,.T.);
#1935=FACE_OUTER_BOUND('',#2788,.T.);
#1936=FACE_OUTER_BOUND('',#2789,.T.);
#1937=FACE_OUTER_BOUND('',#2790,.T.);
#1938=FACE_OUTER_BOUND('',#2791,.T.);
#1939=FACE_OUTER_BOUND('',#2792,.T.);
#1940=FACE_OUTER_BOUND('',#2793,.T.);
#1941=FACE_OUTER_BOUND('',#2794,.T.);
#1942=FACE_OUTER_BOUND('',#2795,.T.);
#1943=FACE_OUTER_BOUND('',#2796,.T.);
#1944=FACE_OUTER_BOUND('',#2797,.T.);
#1945=FACE_OUTER_BOUND('',#2798,.T.);
#1946=FACE_OUTER_BOUND('',#2799,.T.);
#1947=FACE_OUTER_BOUND('',#2800,.T.);
#2719=EDGE_LOOP('',(#11699,#11700,#11701,#11702,#11703,#11704));
#2720=EDGE_LOOP('',(#11705,#11706,#11707,#11708));
#2721=EDGE_LOOP('',(#11709,#11710,#11711,#11712));
#2722=EDGE_LOOP('',(#11713,#11714,#11715,#11716));
#2723=EDGE_LOOP('',(#11717,#11718,#11719,#11720));
#2724=EDGE_LOOP('',(#11721,#11722,#11723,#11724));
#2725=EDGE_LOOP('',(#11725,#11726,#11727,#11728));
#2726=EDGE_LOOP('',(#11729,#11730,#11731,#11732));
#2727=EDGE_LOOP('',(#11733,#11734,#11735,#11736,#11737,#11738,#11739,#11740,
#11741,#11742,#11743,#11744,#11745,#11746,#11747,#11748,#11749,#11750,#11751,
#11752,#11753,#11754));
#2728=EDGE_LOOP('',(#11755,#11756,#11757,#11758));
#2729=EDGE_LOOP('',(#11759,#11760,#11761,#11762));
#2730=EDGE_LOOP('',(#11763,#11764,#11765,#11766));
#2731=EDGE_LOOP('',(#11767,#11768,#11769,#11770));
#2732=EDGE_LOOP('',(#11771,#11772,#11773));
#2733=EDGE_LOOP('',(#11774,#11775,#11776,#11777,#11778));
#2734=EDGE_LOOP('',(#11779,#11780,#11781,#11782,#11783));
#2735=EDGE_LOOP('',(#11784,#11785,#11786,#11787));
#2736=EDGE_LOOP('',(#11788,#11789,#11790,#11791));
#2737=EDGE_LOOP('',(#11792,#11793,#11794,#11795,#11796));
#2738=EDGE_LOOP('',(#11797,#11798,#11799,#11800,#11801));
#2739=EDGE_LOOP('',(#11802,#11803,#11804,#11805));
#2740=EDGE_LOOP('',(#11806,#11807,#11808,#11809));
#2741=EDGE_LOOP('',(#11810,#11811,#11812,#11813));
#2742=EDGE_LOOP('',(#11814,#11815,#11816,#11817));
#2743=EDGE_LOOP('',(#11818,#11819,#11820,#11821));
#2744=EDGE_LOOP('',(#11822,#11823,#11824,#11825));
#2745=EDGE_LOOP('',(#11826,#11827,#11828,#11829));
#2746=EDGE_LOOP('',(#11830,#11831,#11832,#11833));
#2747=EDGE_LOOP('',(#11834,#11835,#11836,#11837,#11838,#11839));
#2748=EDGE_LOOP('',(#11840,#11841,#11842,#11843,#11844,#11845));
#2749=EDGE_LOOP('',(#11846,#11847,#11848,#11849,#11850,#11851,#11852,#11853,
#11854,#11855));
#2750=EDGE_LOOP('',(#11856,#11857,#11858,#11859));
#2751=EDGE_LOOP('',(#11860,#11861,#11862,#11863));
#2752=EDGE_LOOP('',(#11864,#11865,#11866,#11867));
#2753=EDGE_LOOP('',(#11868,#11869,#11870,#11871));
#2754=EDGE_LOOP('',(#11872,#11873,#11874,#11875));
#2755=EDGE_LOOP('',(#11876,#11877,#11878,#11879));
#2756=EDGE_LOOP('',(#11880,#11881,#11882,#11883));
#2757=EDGE_LOOP('',(#11884,#11885,#11886,#11887,#11888,#11889,#11890,#11891,
#11892,#11893,#11894,#11895,#11896,#11897,#11898,#11899));
#2758=EDGE_LOOP('',(#11900,#11901,#11902));
#2759=EDGE_LOOP('',(#11903,#11904,#11905,#11906,#11907));
#2760=EDGE_LOOP('',(#11908,#11909,#11910,#11911));
#2761=EDGE_LOOP('',(#11912,#11913,#11914,#11915));
#2762=EDGE_LOOP('',(#11916,#11917,#11918,#11919));
#2763=EDGE_LOOP('',(#11920,#11921,#11922,#11923));
#2764=EDGE_LOOP('',(#11924,#11925,#11926,#11927));
#2765=EDGE_LOOP('',(#11928,#11929,#11930,#11931));
#2766=EDGE_LOOP('',(#11932,#11933,#11934,#11935));
#2767=EDGE_LOOP('',(#11936,#11937,#11938,#11939));
#2768=EDGE_LOOP('',(#11940,#11941,#11942,#11943));
#2769=EDGE_LOOP('',(#11944,#11945,#11946,#11947,#11948));
#2770=EDGE_LOOP('',(#11949,#11950,#11951,#11952));
#2771=EDGE_LOOP('',(#11953,#11954,#11955,#11956,#11957,#11958,#11959,#11960,
#11961,#11962));
#2772=EDGE_LOOP('',(#11963,#11964,#11965,#11966,#11967,#11968));
#2773=EDGE_LOOP('',(#11969,#11970,#11971,#11972,#11973,#11974,#11975,#11976,
#11977,#11978));
#2774=EDGE_LOOP('',(#11979,#11980,#11981,#11982));
#2775=EDGE_LOOP('',(#11983,#11984,#11985,#11986));
#2776=EDGE_LOOP('',(#11987,#11988,#11989,#11990));
#2777=EDGE_LOOP('',(#11991,#11992,#11993,#11994));
#2778=EDGE_LOOP('',(#11995,#11996,#11997,#11998));
#2779=EDGE_LOOP('',(#11999,#12000,#12001,#12002));
#2780=EDGE_LOOP('',(#12003,#12004,#12005,#12006));
#2781=EDGE_LOOP('',(#12007,#12008,#12009,#12010));
#2782=EDGE_LOOP('',(#12011,#12012,#12013,#12014));
#2783=EDGE_LOOP('',(#12015,#12016,#12017,#12018,#12019,#12020));
#2784=EDGE_LOOP('',(#12021,#12022,#12023,#12024,#12025,#12026));
#2785=EDGE_LOOP('',(#12027,#12028,#12029,#12030,#12031,#12032,#12033,#12034,
#12035,#12036));
#2786=EDGE_LOOP('',(#12037,#12038,#12039,#12040));
#2787=EDGE_LOOP('',(#12041,#12042,#12043,#12044));
#2788=EDGE_LOOP('',(#12045,#12046,#12047,#12048));
#2789=EDGE_LOOP('',(#12049,#12050,#12051,#12052));
#2790=EDGE_LOOP('',(#12053,#12054,#12055,#12056));
#2791=EDGE_LOOP('',(#12057,#12058,#12059,#12060));
#2792=EDGE_LOOP('',(#12061,#12062,#12063,#12064));
#2793=EDGE_LOOP('',(#12065,#12066,#12067,#12068,#12069,#12070));
#2794=EDGE_LOOP('',(#12071,#12072,#12073,#12074,#12075,#12076));
#2795=EDGE_LOOP('',(#12077,#12078,#12079,#12080,#12081,#12082,#12083,#12084,
#12085,#12086));
#2796=EDGE_LOOP('',(#12087,#12088,#12089,#12090));
#2797=EDGE_LOOP('',(#12091,#12092,#12093,#12094));
#2798=EDGE_LOOP('',(#12095,#12096,#12097,#12098));
#2799=EDGE_LOOP('',(#12099,#12100,#12101,#12102));
#2800=EDGE_LOOP('',(#12103,#12104,#12105,#12106,#12107,#12108,#12109,#12110));
#3842=LINE('',#29370,#5153);
#3843=LINE('',#29372,#5154);
#3844=LINE('',#29374,#5155);
#3845=LINE('',#29376,#5156);
#3846=LINE('',#29378,#5157);
#3847=LINE('',#29379,#5158);
#3848=LINE('',#29383,#5159);
#3849=LINE('',#29389,#5160);
#3850=LINE('',#29390,#5161);
#3851=LINE('',#29391,#5162);
#3852=LINE('',#29395,#5163);
#3853=LINE('',#29401,#5164);
#3854=LINE('',#29402,#5165);
#3855=LINE('',#29403,#5166);
#3856=LINE('',#29407,#5167);
#3857=LINE('',#29413,#5168);
#3858=LINE('',#29414,#5169);
#3859=LINE('',#29415,#5170);
#3860=LINE('',#29421,#5171);
#3861=LINE('',#29423,#5172);
#3862=LINE('',#29425,#5173);
#3863=LINE('',#29429,#5174);
#3864=LINE('',#29433,#5175);
#3865=LINE('',#29437,#5176);
#3866=LINE('',#29441,#5177);
#3867=LINE('',#29443,#5178);
#3868=LINE('',#29444,#5179);
#3869=LINE('',#29447,#5180);
#3870=LINE('',#29450,#5181);
#3871=LINE('',#29453,#5182);
#3872=LINE('',#29454,#5183);
#3873=LINE('',#29457,#5184);
#3874=LINE('',#29461,#5185);
#3875=LINE('',#29462,#5186);
#3876=LINE('',#29466,#5187);
#3877=LINE('',#29468,#5188);
#3878=LINE('',#29469,#5189);
#3879=LINE('',#29473,#5190);
#3880=LINE('',#29474,#5191);
#3881=LINE('',#29476,#5192);
#3882=LINE('',#29477,#5193);
#3883=LINE('',#29481,#5194);
#3884=LINE('',#29482,#5195);
#3885=LINE('',#29484,#5196);
#3886=LINE('',#29485,#5197);
#3887=LINE('',#29487,#5198);
#3888=LINE('',#29488,#5199);
#3889=LINE('',#29491,#5200);
#3890=LINE('',#29492,#5201);
#3891=LINE('',#29495,#5202);
#3892=LINE('',#29497,#5203);
#3893=LINE('',#29498,#5204);
#3894=LINE('',#29500,#5205);
#3895=LINE('',#29501,#5206);
#3896=LINE('',#29707,#5207);
#3897=LINE('',#29912,#5208);
#3898=LINE('',#29940,#5209);
#3899=LINE('',#29949,#5210);
#3900=LINE('',#29953,#5211);
#3901=LINE('',#30006,#5212);
#3902=LINE('',#30038,#5213);
#3903=LINE('',#30140,#5214);
#3904=LINE('',#30143,#5215);
#3905=LINE('',#30145,#5216);
#3906=LINE('',#30147,#5217);
#3907=LINE('',#30148,#5218);
#3908=LINE('',#30151,#5219);
#3909=LINE('',#30365,#5220);
#3910=LINE('',#30499,#5221);
#3911=LINE('',#30503,#5222);
#3912=LINE('',#30507,#5223);
#3913=LINE('',#30560,#5224);
#3914=LINE('',#30592,#5225);
#3915=LINE('',#30606,#5226);
#3916=LINE('',#30619,#5227);
#3917=LINE('',#30622,#5228);
#3918=LINE('',#30623,#5229);
#3919=LINE('',#30626,#5230);
#3920=LINE('',#30627,#5231);
#3921=LINE('',#30631,#5232);
#3922=LINE('',#30632,#5233);
#3923=LINE('',#30633,#5234);
#3924=LINE('',#30636,#5235);
#3925=LINE('',#30640,#5236);
#3926=LINE('',#30641,#5237);
#3927=LINE('',#30643,#5238);
#3928=LINE('',#30646,#5239);
#3929=LINE('',#30648,#5240);
#3930=LINE('',#30651,#5241);
#3931=LINE('',#30652,#5242);
#3932=LINE('',#30655,#5243);
#3933=LINE('',#30659,#5244);
#3934=LINE('',#30660,#5245);
#3935=LINE('',#30662,#5246);
#3936=LINE('',#30663,#5247);
#3937=LINE('',#30665,#5248);
#3938=LINE('',#30666,#5249);
#3939=LINE('',#30668,#5250);
#3940=LINE('',#30671,#5251);
#3941=LINE('',#30673,#5252);
#3942=LINE('',#30674,#5253);
#3943=LINE('',#30677,#5254);
#3944=LINE('',#31064,#5255);
#3945=LINE('',#31269,#5256);
#3946=LINE('',#31296,#5257);
#3947=LINE('',#31304,#5258);
#3948=LINE('',#31307,#5259);
#3949=LINE('',#31354,#5260);
#3950=LINE('',#31381,#5261);
#3951=LINE('',#31383,#5262);
#3952=LINE('',#31385,#5263);
#3953=LINE('',#31526,#5264);
#3954=LINE('',#31678,#5265);
#3955=LINE('',#31685,#5266);
#3956=LINE('',#31686,#5267);
#3957=LINE('',#31728,#5268);
#3958=LINE('',#31747,#5269);
#3959=LINE('',#31751,#5270);
#3960=LINE('',#31755,#5271);
#3961=LINE('',#31756,#5272);
#3962=LINE('',#31759,#5273);
#3963=LINE('',#31762,#5274);
#5153=VECTOR('',#17612,10.);
#5154=VECTOR('',#17613,10.);
#5155=VECTOR('',#17614,10.);
#5156=VECTOR('',#17615,10.);
#5157=VECTOR('',#17616,10.);
#5158=VECTOR('',#17617,10.);
#5159=VECTOR('',#17620,10.);
#5160=VECTOR('',#17627,10.);
#5161=VECTOR('',#17628,10.);
#5162=VECTOR('',#17629,10.);
#5163=VECTOR('',#17632,10.);
#5164=VECTOR('',#17639,10.);
#5165=VECTOR('',#17640,10.);
#5166=VECTOR('',#17641,10.);
#5167=VECTOR('',#17644,10.);
#5168=VECTOR('',#17651,10.);
#5169=VECTOR('',#17652,10.);
#5170=VECTOR('',#17653,10.);
#5171=VECTOR('',#17662,10.);
#5172=VECTOR('',#17663,10.);
#5173=VECTOR('',#17664,10.);
#5174=VECTOR('',#17667,10.);
#5175=VECTOR('',#17670,10.);
#5176=VECTOR('',#17673,10.);
#5177=VECTOR('',#17676,10.);
#5178=VECTOR('',#17677,10.);
#5179=VECTOR('',#17678,10.);
#5180=VECTOR('',#17681,10.);
#5181=VECTOR('',#17684,10.);
#5182=VECTOR('',#17687,10.);
#5183=VECTOR('',#17688,10.);
#5184=VECTOR('',#17691,10.);
#5185=VECTOR('',#17696,10.);
#5186=VECTOR('',#17697,10.);
#5187=VECTOR('',#17700,10.);
#5188=VECTOR('',#17701,10.);
#5189=VECTOR('',#17702,10.);
#5190=VECTOR('',#17705,10.);
#5191=VECTOR('',#17706,10.);
#5192=VECTOR('',#17707,10.);
#5193=VECTOR('',#17708,10.);
#5194=VECTOR('',#17711,10.);
#5195=VECTOR('',#17712,10.);
#5196=VECTOR('',#17713,10.);
#5197=VECTOR('',#17714,10.);
#5198=VECTOR('',#17717,10.);
#5199=VECTOR('',#17718,10.);
#5200=VECTOR('',#17721,10.);
#5201=VECTOR('',#17722,10.);
#5202=VECTOR('',#17725,10.);
#5203=VECTOR('',#17726,10.);
#5204=VECTOR('',#17727,10.);
#5205=VECTOR('',#17730,10.);
#5206=VECTOR('',#17731,10.);
#5207=VECTOR('',#17734,10.);
#5208=VECTOR('',#17735,10.);
#5209=VECTOR('',#17736,10.);
#5210=VECTOR('',#17739,10.);
#5211=VECTOR('',#17742,10.);
#5212=VECTOR('',#17745,10.);
#5213=VECTOR('',#17748,10.);
#5214=VECTOR('',#17749,10.);
#5215=VECTOR('',#17752,10.);
#5216=VECTOR('',#17753,10.);
#5217=VECTOR('',#17754,10.);
#5218=VECTOR('',#17755,10.);
#5219=VECTOR('',#17758,10.);
#5220=VECTOR('',#17761,10.);
#5221=VECTOR('',#17762,10.);
#5222=VECTOR('',#17765,10.);
#5223=VECTOR('',#17768,10.);
#5224=VECTOR('',#17771,10.);
#5225=VECTOR('',#17774,10.);
#5226=VECTOR('',#17777,10.);
#5227=VECTOR('',#17780,10.);
#5228=VECTOR('',#17783,10.);
#5229=VECTOR('',#17784,10.);
#5230=VECTOR('',#17787,10.);
#5231=VECTOR('',#17788,10.);
#5232=VECTOR('',#17791,10.);
#5233=VECTOR('',#17792,10.);
#5234=VECTOR('',#17793,10.);
#5235=VECTOR('',#17796,10.);
#5236=VECTOR('',#17801,10.);
#5237=VECTOR('',#17802,10.);
#5238=VECTOR('',#17805,10.);
#5239=VECTOR('',#17810,10.);
#5240=VECTOR('',#17813,10.);
#5241=VECTOR('',#17816,10.);
#5242=VECTOR('',#17817,10.);
#5243=VECTOR('',#17820,10.);
#5244=VECTOR('',#17825,10.);
#5245=VECTOR('',#17826,10.);
#5246=VECTOR('',#17829,10.);
#5247=VECTOR('',#17830,10.);
#5248=VECTOR('',#17833,10.);
#5249=VECTOR('',#17834,10.);
#5250=VECTOR('',#17837,10.);
#5251=VECTOR('',#17840,10.);
#5252=VECTOR('',#17841,10.);
#5253=VECTOR('',#17842,10.);
#5254=VECTOR('',#17845,10.);
#5255=VECTOR('',#17852,10.);
#5256=VECTOR('',#17853,10.);
#5257=VECTOR('',#17854,10.);
#5258=VECTOR('',#17857,10.);
#5259=VECTOR('',#17860,10.);
#5260=VECTOR('',#17861,10.);
#5261=VECTOR('',#17864,10.);
#5262=VECTOR('',#17867,10.);
#5263=VECTOR('',#17870,10.);
#5264=VECTOR('',#17871,10.);
#5265=VECTOR('',#17872,10.);
#5266=VECTOR('',#17875,10.);
#5267=VECTOR('',#17876,10.);
#5268=VECTOR('',#17877,10.);
#5269=VECTOR('',#17882,10.);
#5270=VECTOR('',#17887,10.);
#5271=VECTOR('',#17892,10.);
#5272=VECTOR('',#17893,10.);
#5273=VECTOR('',#17896,10.);
#5274=VECTOR('',#17901,10.);
#6434=VERTEX_POINT('',#29368);
#6435=VERTEX_POINT('',#29369);
#6436=VERTEX_POINT('',#29371);
#6437=VERTEX_POINT('',#29373);
#6438=VERTEX_POINT('',#29375);
#6439=VERTEX_POINT('',#29377);
#6440=VERTEX_POINT('',#29381);
#6441=VERTEX_POINT('',#29382);
#6442=VERTEX_POINT('',#29387);
#6443=VERTEX_POINT('',#29388);
#6444=VERTEX_POINT('',#29393);
#6445=VERTEX_POINT('',#29394);
#6446=VERTEX_POINT('',#29399);
#6447=VERTEX_POINT('',#29400);
#6448=VERTEX_POINT('',#29405);
#6449=VERTEX_POINT('',#29406);
#6450=VERTEX_POINT('',#29411);
#6451=VERTEX_POINT('',#29412);
#6452=VERTEX_POINT('',#29420);
#6453=VERTEX_POINT('',#29422);
#6454=VERTEX_POINT('',#29424);
#6455=VERTEX_POINT('',#29426);
#6456=VERTEX_POINT('',#29428);
#6457=VERTEX_POINT('',#29430);
#6458=VERTEX_POINT('',#29432);
#6459=VERTEX_POINT('',#29434);
#6460=VERTEX_POINT('',#29436);
#6461=VERTEX_POINT('',#29438);
#6462=VERTEX_POINT('',#29440);
#6463=VERTEX_POINT('',#29442);
#6464=VERTEX_POINT('',#29446);
#6465=VERTEX_POINT('',#29448);
#6466=VERTEX_POINT('',#29452);
#6467=VERTEX_POINT('',#29456);
#6468=VERTEX_POINT('',#29460);
#6469=VERTEX_POINT('',#29464);
#6470=VERTEX_POINT('',#29465);
#6471=VERTEX_POINT('',#29467);
#6472=VERTEX_POINT('',#29471);
#6473=VERTEX_POINT('',#29472);
#6474=VERTEX_POINT('',#29475);
#6475=VERTEX_POINT('',#29479);
#6476=VERTEX_POINT('',#29480);
#6477=VERTEX_POINT('',#29483);
#6478=VERTEX_POINT('',#29490);
#6479=VERTEX_POINT('',#29494);
#6480=VERTEX_POINT('',#29496);
#6481=VERTEX_POINT('',#29535);
#6482=VERTEX_POINT('',#29536);
#6483=VERTEX_POINT('',#29631);
#6484=VERTEX_POINT('',#29636);
#6485=VERTEX_POINT('',#29740);
#6486=VERTEX_POINT('',#29741);
#6487=VERTEX_POINT('',#29812);
#6488=VERTEX_POINT('',#29817);
#6489=VERTEX_POINT('',#29933);
#6490=VERTEX_POINT('',#29939);
#6491=VERTEX_POINT('',#29947);
#6492=VERTEX_POINT('',#29948);
#6493=VERTEX_POINT('',#29950);
#6494=VERTEX_POINT('',#29952);
#6495=VERTEX_POINT('',#29999);
#6496=VERTEX_POINT('',#30005);
#6497=VERTEX_POINT('',#30037);
#6498=VERTEX_POINT('',#30039);
#6499=VERTEX_POINT('',#30134);
#6500=VERTEX_POINT('',#30142);
#6501=VERTEX_POINT('',#30144);
#6502=VERTEX_POINT('',#30146);
#6503=VERTEX_POINT('',#30150);
#6504=VERTEX_POINT('',#30193);
#6505=VERTEX_POINT('',#30194);
#6506=VERTEX_POINT('',#30289);
#6507=VERTEX_POINT('',#30294);
#6508=VERTEX_POINT('',#30398);
#6509=VERTEX_POINT('',#30493);
#6510=VERTEX_POINT('',#30501);
#6511=VERTEX_POINT('',#30502);
#6512=VERTEX_POINT('',#30504);
#6513=VERTEX_POINT('',#30506);
#6514=VERTEX_POINT('',#30553);
#6515=VERTEX_POINT('',#30559);
#6516=VERTEX_POINT('',#30591);
#6517=VERTEX_POINT('',#30593);
#6518=VERTEX_POINT('',#30598);
#6519=VERTEX_POINT('',#30600);
#6520=VERTEX_POINT('',#30605);
#6521=VERTEX_POINT('',#30607);
#6522=VERTEX_POINT('',#30612);
#6523=VERTEX_POINT('',#30614);
#6524=VERTEX_POINT('',#30621);
#6525=VERTEX_POINT('',#30625);
#6526=VERTEX_POINT('',#30629);
#6527=VERTEX_POINT('',#30630);
#6528=VERTEX_POINT('',#30635);
#6529=VERTEX_POINT('',#30639);
#6530=VERTEX_POINT('',#30650);
#6531=VERTEX_POINT('',#30654);
#6532=VERTEX_POINT('',#30658);
#6533=VERTEX_POINT('',#30670);
#6534=VERTEX_POINT('',#30672);
#6535=VERTEX_POINT('',#30676);
#6536=VERTEX_POINT('',#30678);
#6537=VERTEX_POINT('',#30749);
#6538=VERTEX_POINT('',#30755);
#6539=VERTEX_POINT('',#30760);
#6540=VERTEX_POINT('',#30762);
#6541=VERTEX_POINT('',#30767);
#6542=VERTEX_POINT('',#30892);
#6543=VERTEX_POINT('',#30893);
#6544=VERTEX_POINT('',#30988);
#6545=VERTEX_POINT('',#30993);
#6546=VERTEX_POINT('',#31097);
#6547=VERTEX_POINT('',#31098);
#6548=VERTEX_POINT('',#31169);
#6549=VERTEX_POINT('',#31174);
#6550=VERTEX_POINT('',#31290);
#6551=VERTEX_POINT('',#31303);
#6552=VERTEX_POINT('',#31305);
#6553=VERTEX_POINT('',#31353);
#6554=VERTEX_POINT('',#31426);
#6555=VERTEX_POINT('',#31427);
#6556=VERTEX_POINT('',#31559);
#6557=VERTEX_POINT('',#31750);
#6558=VERTEX_POINT('',#31754);
#6559=VERTEX_POINT('',#31758);
#8226=EDGE_CURVE('',#6434,#6435,#3842,.T.);
#8227=EDGE_CURVE('',#6435,#6436,#3843,.T.);
#8228=EDGE_CURVE('',#6436,#6437,#3844,.T.);
#8229=EDGE_CURVE('',#6437,#6438,#3845,.T.);
#8230=EDGE_CURVE('',#6438,#6439,#3846,.T.);
#8231=EDGE_CURVE('',#6439,#6434,#3847,.T.);
#8232=EDGE_CURVE('',#6440,#6441,#3848,.T.);
#8233=EDGE_CURVE('',#6441,#6435,#1065,.T.);
#8234=EDGE_CURVE('',#6434,#6440,#1066,.T.);
#8235=EDGE_CURVE('',#6442,#6443,#3849,.T.);
#8236=EDGE_CURVE('',#6443,#6441,#3850,.T.);
#8237=EDGE_CURVE('',#6440,#6442,#3851,.T.);
#8238=EDGE_CURVE('',#6444,#6445,#3852,.T.);
#8239=EDGE_CURVE('',#6445,#6443,#1067,.T.);
#8240=EDGE_CURVE('',#6442,#6444,#1068,.T.);
#8241=EDGE_CURVE('',#6446,#6447,#3853,.T.);
#8242=EDGE_CURVE('',#6447,#6445,#3854,.T.);
#8243=EDGE_CURVE('',#6444,#6446,#3855,.T.);
#8244=EDGE_CURVE('',#6448,#6449,#3856,.T.);
#8245=EDGE_CURVE('',#6449,#6447,#1069,.T.);
#8246=EDGE_CURVE('',#6446,#6448,#1070,.T.);
#8247=EDGE_CURVE('',#6450,#6451,#3857,.T.);
#8248=EDGE_CURVE('',#6451,#6449,#3858,.T.);
#8249=EDGE_CURVE('',#6448,#6450,#3859,.T.);
#8250=EDGE_CURVE('',#6438,#6451,#1071,.T.);
#8251=EDGE_CURVE('',#6450,#6439,#1072,.T.);
#8252=EDGE_CURVE('',#6452,#6437,#3860,.F.);
#8253=EDGE_CURVE('',#6452,#6453,#3861,.T.);
#8254=EDGE_CURVE('',#6454,#6453,#3862,.T.);
#8255=EDGE_CURVE('',#6455,#6454,#1073,.T.);
#8256=EDGE_CURVE('',#6456,#6455,#3863,.T.);
#8257=EDGE_CURVE('',#6457,#6456,#1074,.T.);
#8258=EDGE_CURVE('',#6458,#6457,#3864,.T.);
#8259=EDGE_CURVE('',#6459,#6458,#1075,.T.);
#8260=EDGE_CURVE('',#6460,#6459,#3865,.T.);
#8261=EDGE_CURVE('',#6461,#6460,#1076,.T.);
#8262=EDGE_CURVE('',#6462,#6461,#3866,.T.);
#8263=EDGE_CURVE('',#6462,#6463,#3867,.T.);
#8264=EDGE_CURVE('',#6436,#6463,#3868,.F.);
#8265=EDGE_CURVE('',#6442,#6464,#3869,.T.);
#8266=EDGE_CURVE('',#6464,#6465,#1077,.T.);
#8267=EDGE_CURVE('',#6444,#6465,#3870,.T.);
#8268=EDGE_CURVE('',#6440,#6466,#3871,.T.);
#8269=EDGE_CURVE('',#6466,#6464,#3872,.T.);
#8270=EDGE_CURVE('',#6434,#6467,#3873,.T.);
#8271=EDGE_CURVE('',#6467,#6466,#1078,.T.);
#8272=EDGE_CURVE('',#6439,#6468,#3874,.T.);
#8273=EDGE_CURVE('',#6468,#6467,#3875,.T.);
#8274=EDGE_CURVE('',#6469,#6470,#3876,.T.);
#8275=EDGE_CURVE('',#6471,#6469,#3877,.T.);
#8276=EDGE_CURVE('',#6470,#6471,#3878,.T.);
#8277=EDGE_CURVE('',#6472,#6473,#3879,.T.);
#8278=EDGE_CURVE('',#6473,#6471,#3880,.T.);
#8279=EDGE_CURVE('',#6469,#6474,#3881,.T.);
#8280=EDGE_CURVE('',#6474,#6472,#3882,.T.);
#8281=EDGE_CURVE('',#6475,#6476,#3883,.T.);
#8282=EDGE_CURVE('',#6476,#6470,#3884,.T.);
#8283=EDGE_CURVE('',#6471,#6477,#3885,.T.);
#8284=EDGE_CURVE('',#6477,#6475,#3886,.T.);
#8285=EDGE_CURVE('',#6437,#6469,#3887,.T.);
#8286=EDGE_CURVE('',#6470,#6452,#3888,.T.);
#8287=EDGE_CURVE('',#6478,#6473,#3889,.T.);
#8288=EDGE_CURVE('',#6477,#6478,#3890,.T.);
#8289=EDGE_CURVE('',#6479,#6472,#3891,.T.);
#8290=EDGE_CURVE('',#6479,#6480,#3892,.T.);
#8291=EDGE_CURVE('',#6480,#6478,#3893,.T.);
#8292=EDGE_CURVE('',#6474,#6436,#3894,.T.);
#8293=EDGE_CURVE('',#6463,#6479,#3895,.T.);
#8294=EDGE_CURVE('',#6481,#6482,#352,.T.);
#8295=EDGE_CURVE('',#6483,#6482,#353,.T.);
#8296=EDGE_CURVE('',#6483,#6484,#354,.T.);
#8297=EDGE_CURVE('',#6484,#6481,#3896,.T.);
#8298=EDGE_CURVE('',#6485,#6486,#355,.T.);
#8299=EDGE_CURVE('',#6487,#6486,#356,.T.);
#8300=EDGE_CURVE('',#6487,#6488,#357,.T.);
#8301=EDGE_CURVE('',#6488,#6485,#3897,.T.);
#8302=EDGE_CURVE('',#6486,#6489,#358,.T.);
#8303=EDGE_CURVE('',#6489,#6490,#3898,.T.);
#8304=EDGE_CURVE('',#6490,#6487,#359,.T.);
#8305=EDGE_CURVE('',#6491,#6492,#3899,.T.);
#8306=EDGE_CURVE('',#6492,#6493,#1079,.T.);
#8307=EDGE_CURVE('',#6493,#6494,#3900,.T.);
#8308=EDGE_CURVE('',#6494,#6491,#1080,.T.);
#8309=EDGE_CURVE('',#6491,#6490,#360,.T.);
#8310=EDGE_CURVE('',#6489,#6492,#361,.T.);
#8311=EDGE_CURVE('',#6482,#6495,#362,.T.);
#8312=EDGE_CURVE('',#6495,#6496,#3901,.T.);
#8313=EDGE_CURVE('',#6496,#6483,#363,.T.);
#8314=EDGE_CURVE('',#6495,#6494,#364,.T.);
#8315=EDGE_CURVE('',#6493,#6496,#365,.T.);
#8316=EDGE_CURVE('',#6481,#6497,#3902,.T.);
#8317=EDGE_CURVE('',#6498,#6497,#366,.T.);
#8318=EDGE_CURVE('',#6499,#6498,#367,.T.);
#8319=EDGE_CURVE('',#6499,#6495,#3903,.T.);
#8320=EDGE_CURVE('',#6484,#6500,#3904,.T.);
#8321=EDGE_CURVE('',#6501,#6500,#3905,.T.);
#8322=EDGE_CURVE('',#6502,#6501,#3906,.T.);
#8323=EDGE_CURVE('',#6497,#6502,#3907,.T.);
#8324=EDGE_CURVE('',#6485,#6503,#3908,.T.);
#8325=EDGE_CURVE('',#6500,#6503,#1081,.T.);
#8326=EDGE_CURVE('',#6504,#6505,#368,.T.);
#8327=EDGE_CURVE('',#6506,#6505,#369,.T.);
#8328=EDGE_CURVE('',#6506,#6507,#370,.T.);
#8329=EDGE_CURVE('',#6507,#6504,#3909,.T.);
#8330=EDGE_CURVE('',#6502,#6508,#371,.T.);
#8331=EDGE_CURVE('',#6498,#6508,#372,.T.);
#8332=EDGE_CURVE('',#6508,#6509,#373,.T.);
#8333=EDGE_CURVE('',#6509,#6499,#3910,.T.);
#8334=EDGE_CURVE('',#6510,#6511,#3911,.T.);
#8335=EDGE_CURVE('',#6511,#6512,#1082,.T.);
#8336=EDGE_CURVE('',#6512,#6513,#3912,.T.);
#8337=EDGE_CURVE('',#6513,#6510,#1083,.T.);
#8338=EDGE_CURVE('',#6510,#6499,#374,.T.);
#8339=EDGE_CURVE('',#6509,#6511,#375,.T.);
#8340=EDGE_CURVE('',#6505,#6514,#376,.T.);
#8341=EDGE_CURVE('',#6514,#6515,#3913,.T.);
#8342=EDGE_CURVE('',#6515,#6506,#377,.T.);
#8343=EDGE_CURVE('',#6514,#6513,#378,.T.);
#8344=EDGE_CURVE('',#6512,#6515,#379,.T.);
#8345=EDGE_CURVE('',#6516,#6514,#3914,.T.);
#8346=EDGE_CURVE('',#6517,#6516,#380,.T.);
#8347=EDGE_CURVE('',#6518,#6517,#1084,.T.);
#8348=EDGE_CURVE('',#6519,#6518,#381,.T.);
#8349=EDGE_CURVE('',#6520,#6519,#3915,.T.);
#8350=EDGE_CURVE('',#6521,#6520,#382,.T.);
#8351=EDGE_CURVE('',#6522,#6521,#1085,.T.);
#8352=EDGE_CURVE('',#6523,#6522,#383,.T.);
#8353=EDGE_CURVE('',#6490,#6523,#3916,.T.);
#8354=EDGE_CURVE('',#6478,#6524,#3917,.T.);
#8355=EDGE_CURVE('',#6524,#6480,#3918,.T.);
#8356=EDGE_CURVE('',#6524,#6525,#3919,.T.);
#8357=EDGE_CURVE('',#6525,#6475,#3920,.T.);
#8358=EDGE_CURVE('',#6526,#6527,#3921,.T.);
#8359=EDGE_CURVE('',#6527,#6454,#3922,.T.);
#8360=EDGE_CURVE('',#6453,#6526,#3923,.T.);
#8361=EDGE_CURVE('',#6528,#6455,#3924,.T.);
#8362=EDGE_CURVE('',#6527,#6528,#1086,.T.);
#8363=EDGE_CURVE('',#6529,#6456,#3925,.T.);
#8364=EDGE_CURVE('',#6528,#6529,#3926,.T.);
#8365=EDGE_CURVE('',#6501,#6457,#3927,.T.);
#8366=EDGE_CURVE('',#6529,#6501,#1087,.T.);
#8367=EDGE_CURVE('',#6500,#6458,#3928,.T.);
#8368=EDGE_CURVE('',#6503,#6459,#3929,.T.);
#8369=EDGE_CURVE('',#6530,#6460,#3930,.T.);
#8370=EDGE_CURVE('',#6503,#6530,#3931,.T.);
#8371=EDGE_CURVE('',#6531,#6461,#3932,.T.);
#8372=EDGE_CURVE('',#6530,#6531,#1088,.T.);
#8373=EDGE_CURVE('',#6531,#6532,#3933,.T.);
#8374=EDGE_CURVE('',#6532,#6462,#3934,.T.);
#8375=EDGE_CURVE('',#6525,#6526,#3935,.T.);
#8376=EDGE_CURVE('',#6453,#6476,#3936,.T.);
#8377=EDGE_CURVE('',#6532,#6524,#3937,.T.);
#8378=EDGE_CURVE('',#6480,#6462,#3938,.T.);
#8379=EDGE_CURVE('',#6507,#6529,#3939,.T.);
#8380=EDGE_CURVE('',#6533,#6528,#3940,.T.);
#8381=EDGE_CURVE('',#6534,#6533,#3941,.T.);
#8382=EDGE_CURVE('',#6504,#6534,#3942,.T.);
#8383=EDGE_CURVE('',#6535,#6527,#3943,.T.);
#8384=EDGE_CURVE('',#6536,#6535,#384,.T.);
#8385=EDGE_CURVE('',#6537,#6536,#385,.T.);
#8386=EDGE_CURVE('',#6538,#6537,#386,.T.);
#8387=EDGE_CURVE('',#6539,#6538,#1089,.T.);
#8388=EDGE_CURVE('',#6540,#6539,#387,.T.);
#8389=EDGE_CURVE('',#6541,#6540,#87,.T.);
#8390=EDGE_CURVE('',#6533,#6541,#388,.T.);
#8391=EDGE_CURVE('',#6542,#6543,#389,.T.);
#8392=EDGE_CURVE('',#6544,#6543,#390,.T.);
#8393=EDGE_CURVE('',#6544,#6545,#391,.T.);
#8394=EDGE_CURVE('',#6545,#6542,#3944,.T.);
#8395=EDGE_CURVE('',#6546,#6547,#392,.T.);
#8396=EDGE_CURVE('',#6548,#6547,#393,.T.);
#8397=EDGE_CURVE('',#6548,#6549,#394,.T.);
#8398=EDGE_CURVE('',#6549,#6546,#3945,.T.);
#8399=EDGE_CURVE('',#6547,#6550,#395,.T.);
#8400=EDGE_CURVE('',#6550,#6520,#3946,.T.);
#8401=EDGE_CURVE('',#6520,#6548,#396,.T.);
#8402=EDGE_CURVE('',#6521,#6551,#3947,.T.);
#8403=EDGE_CURVE('',#6551,#6552,#1090,.T.);
#8404=EDGE_CURVE('',#6552,#6522,#3948,.T.);
#8405=EDGE_CURVE('',#6550,#6551,#397,.T.);
#8406=EDGE_CURVE('',#6543,#6523,#398,.T.);
#8407=EDGE_CURVE('',#6523,#6553,#3949,.T.);
#8408=EDGE_CURVE('',#6553,#6544,#399,.T.);
#8409=EDGE_CURVE('',#6552,#6553,#400,.T.);
#8410=EDGE_CURVE('',#6542,#6488,#3950,.T.);
#8411=EDGE_CURVE('',#6545,#6530,#3951,.T.);
#8412=EDGE_CURVE('',#6546,#6531,#3952,.T.);
#8413=EDGE_CURVE('',#6554,#6555,#401,.T.);
#8414=EDGE_CURVE('',#6536,#6555,#402,.T.);
#8415=EDGE_CURVE('',#6535,#6554,#3953,.T.);
#8416=EDGE_CURVE('',#6556,#6541,#403,.T.);
#8417=EDGE_CURVE('',#6556,#6534,#404,.T.);
#8418=EDGE_CURVE('',#6540,#6516,#3954,.T.);
#8419=EDGE_CURVE('',#6516,#6556,#405,.T.);
#8420=EDGE_CURVE('',#6517,#6539,#3955,.T.);
#8421=EDGE_CURVE('',#6538,#6518,#3956,.T.);
#8422=EDGE_CURVE('',#6555,#6519,#406,.T.);
#8423=EDGE_CURVE('',#6519,#6537,#3957,.T.);
#8424=EDGE_CURVE('',#6554,#6549,#3958,.T.);
#8425=EDGE_CURVE('',#6450,#6557,#3959,.T.);
#8426=EDGE_CURVE('',#6557,#6468,#1091,.T.);
#8427=EDGE_CURVE('',#6448,#6558,#3960,.T.);
#8428=EDGE_CURVE('',#6558,#6557,#3961,.T.);
#8429=EDGE_CURVE('',#6446,#6559,#3962,.T.);
#8430=EDGE_CURVE('',#6559,#6558,#1092,.T.);
#8431=EDGE_CURVE('',#6465,#6559,#3963,.T.);
#11699=ORIENTED_EDGE('',*,*,#8226,.T.);
#11700=ORIENTED_EDGE('',*,*,#8227,.T.);
#11701=ORIENTED_EDGE('',*,*,#8228,.T.);
#11702=ORIENTED_EDGE('',*,*,#8229,.T.);
#11703=ORIENTED_EDGE('',*,*,#8230,.T.);
#11704=ORIENTED_EDGE('',*,*,#8231,.T.);
#11705=ORIENTED_EDGE('',*,*,#8232,.T.);
#11706=ORIENTED_EDGE('',*,*,#8233,.T.);
#11707=ORIENTED_EDGE('',*,*,#8226,.F.);
#11708=ORIENTED_EDGE('',*,*,#8234,.T.);
#11709=ORIENTED_EDGE('',*,*,#8235,.T.);
#11710=ORIENTED_EDGE('',*,*,#8236,.T.);
#11711=ORIENTED_EDGE('',*,*,#8232,.F.);
#11712=ORIENTED_EDGE('',*,*,#8237,.T.);
#11713=ORIENTED_EDGE('',*,*,#8238,.T.);
#11714=ORIENTED_EDGE('',*,*,#8239,.T.);
#11715=ORIENTED_EDGE('',*,*,#8235,.F.);
#11716=ORIENTED_EDGE('',*,*,#8240,.T.);
#11717=ORIENTED_EDGE('',*,*,#8241,.T.);
#11718=ORIENTED_EDGE('',*,*,#8242,.T.);
#11719=ORIENTED_EDGE('',*,*,#8238,.F.);
#11720=ORIENTED_EDGE('',*,*,#8243,.T.);
#11721=ORIENTED_EDGE('',*,*,#8244,.T.);
#11722=ORIENTED_EDGE('',*,*,#8245,.T.);
#11723=ORIENTED_EDGE('',*,*,#8241,.F.);
#11724=ORIENTED_EDGE('',*,*,#8246,.T.);
#11725=ORIENTED_EDGE('',*,*,#8247,.T.);
#11726=ORIENTED_EDGE('',*,*,#8248,.T.);
#11727=ORIENTED_EDGE('',*,*,#8244,.F.);
#11728=ORIENTED_EDGE('',*,*,#8249,.T.);
#11729=ORIENTED_EDGE('',*,*,#8230,.F.);
#11730=ORIENTED_EDGE('',*,*,#8250,.T.);
#11731=ORIENTED_EDGE('',*,*,#8247,.F.);
#11732=ORIENTED_EDGE('',*,*,#8251,.T.);
#11733=ORIENTED_EDGE('',*,*,#8227,.F.);
#11734=ORIENTED_EDGE('',*,*,#8233,.F.);
#11735=ORIENTED_EDGE('',*,*,#8236,.F.);
#11736=ORIENTED_EDGE('',*,*,#8239,.F.);
#11737=ORIENTED_EDGE('',*,*,#8242,.F.);
#11738=ORIENTED_EDGE('',*,*,#8245,.F.);
#11739=ORIENTED_EDGE('',*,*,#8248,.F.);
#11740=ORIENTED_EDGE('',*,*,#8250,.F.);
#11741=ORIENTED_EDGE('',*,*,#8229,.F.);
#11742=ORIENTED_EDGE('',*,*,#8252,.F.);
#11743=ORIENTED_EDGE('',*,*,#8253,.T.);
#11744=ORIENTED_EDGE('',*,*,#8254,.F.);
#11745=ORIENTED_EDGE('',*,*,#8255,.F.);
#11746=ORIENTED_EDGE('',*,*,#8256,.F.);
#11747=ORIENTED_EDGE('',*,*,#8257,.F.);
#11748=ORIENTED_EDGE('',*,*,#8258,.F.);
#11749=ORIENTED_EDGE('',*,*,#8259,.F.);
#11750=ORIENTED_EDGE('',*,*,#8260,.F.);
#11751=ORIENTED_EDGE('',*,*,#8261,.F.);
#11752=ORIENTED_EDGE('',*,*,#8262,.F.);
#11753=ORIENTED_EDGE('',*,*,#8263,.T.);
#11754=ORIENTED_EDGE('',*,*,#8264,.F.);
#11755=ORIENTED_EDGE('',*,*,#8240,.F.);
#11756=ORIENTED_EDGE('',*,*,#8265,.T.);
#11757=ORIENTED_EDGE('',*,*,#8266,.T.);
#11758=ORIENTED_EDGE('',*,*,#8267,.F.);
#11759=ORIENTED_EDGE('',*,*,#8237,.F.);
#11760=ORIENTED_EDGE('',*,*,#8268,.T.);
#11761=ORIENTED_EDGE('',*,*,#8269,.T.);
#11762=ORIENTED_EDGE('',*,*,#8265,.F.);
#11763=ORIENTED_EDGE('',*,*,#8234,.F.);
#11764=ORIENTED_EDGE('',*,*,#8270,.T.);
#11765=ORIENTED_EDGE('',*,*,#8271,.T.);
#11766=ORIENTED_EDGE('',*,*,#8268,.F.);
#11767=ORIENTED_EDGE('',*,*,#8231,.F.);
#11768=ORIENTED_EDGE('',*,*,#8272,.T.);
#11769=ORIENTED_EDGE('',*,*,#8273,.T.);
#11770=ORIENTED_EDGE('',*,*,#8270,.F.);
#11771=ORIENTED_EDGE('',*,*,#8274,.F.);
#11772=ORIENTED_EDGE('',*,*,#8275,.F.);
#11773=ORIENTED_EDGE('',*,*,#8276,.F.);
#11774=ORIENTED_EDGE('',*,*,#8277,.T.);
#11775=ORIENTED_EDGE('',*,*,#8278,.T.);
#11776=ORIENTED_EDGE('',*,*,#8275,.T.);
#11777=ORIENTED_EDGE('',*,*,#8279,.T.);
#11778=ORIENTED_EDGE('',*,*,#8280,.T.);
#11779=ORIENTED_EDGE('',*,*,#8281,.T.);
#11780=ORIENTED_EDGE('',*,*,#8282,.T.);
#11781=ORIENTED_EDGE('',*,*,#8276,.T.);
#11782=ORIENTED_EDGE('',*,*,#8283,.T.);
#11783=ORIENTED_EDGE('',*,*,#8284,.T.);
#11784=ORIENTED_EDGE('',*,*,#8252,.T.);
#11785=ORIENTED_EDGE('',*,*,#8285,.T.);
#11786=ORIENTED_EDGE('',*,*,#8274,.T.);
#11787=ORIENTED_EDGE('',*,*,#8286,.T.);
#11788=ORIENTED_EDGE('',*,*,#8283,.F.);
#11789=ORIENTED_EDGE('',*,*,#8278,.F.);
#11790=ORIENTED_EDGE('',*,*,#8287,.F.);
#11791=ORIENTED_EDGE('',*,*,#8288,.F.);
#11792=ORIENTED_EDGE('',*,*,#8277,.F.);
#11793=ORIENTED_EDGE('',*,*,#8289,.F.);
#11794=ORIENTED_EDGE('',*,*,#8290,.T.);
#11795=ORIENTED_EDGE('',*,*,#8291,.T.);
#11796=ORIENTED_EDGE('',*,*,#8287,.T.);
#11797=ORIENTED_EDGE('',*,*,#8280,.F.);
#11798=ORIENTED_EDGE('',*,*,#8292,.T.);
#11799=ORIENTED_EDGE('',*,*,#8264,.T.);
#11800=ORIENTED_EDGE('',*,*,#8293,.T.);
#11801=ORIENTED_EDGE('',*,*,#8289,.T.);
#11802=ORIENTED_EDGE('',*,*,#8279,.F.);
#11803=ORIENTED_EDGE('',*,*,#8285,.F.);
#11804=ORIENTED_EDGE('',*,*,#8228,.F.);
#11805=ORIENTED_EDGE('',*,*,#8292,.F.);
#11806=ORIENTED_EDGE('',*,*,#8294,.T.);
#11807=ORIENTED_EDGE('',*,*,#8295,.F.);
#11808=ORIENTED_EDGE('',*,*,#8296,.T.);
#11809=ORIENTED_EDGE('',*,*,#8297,.T.);
#11810=ORIENTED_EDGE('',*,*,#8298,.T.);
#11811=ORIENTED_EDGE('',*,*,#8299,.F.);
#11812=ORIENTED_EDGE('',*,*,#8300,.T.);
#11813=ORIENTED_EDGE('',*,*,#8301,.T.);
#11814=ORIENTED_EDGE('',*,*,#8299,.T.);
#11815=ORIENTED_EDGE('',*,*,#8302,.T.);
#11816=ORIENTED_EDGE('',*,*,#8303,.T.);
#11817=ORIENTED_EDGE('',*,*,#8304,.T.);
#11818=ORIENTED_EDGE('',*,*,#8305,.T.);
#11819=ORIENTED_EDGE('',*,*,#8306,.T.);
#11820=ORIENTED_EDGE('',*,*,#8307,.T.);
#11821=ORIENTED_EDGE('',*,*,#8308,.T.);
#11822=ORIENTED_EDGE('',*,*,#8305,.F.);
#11823=ORIENTED_EDGE('',*,*,#8309,.T.);
#11824=ORIENTED_EDGE('',*,*,#8303,.F.);
#11825=ORIENTED_EDGE('',*,*,#8310,.T.);
#11826=ORIENTED_EDGE('',*,*,#8295,.T.);
#11827=ORIENTED_EDGE('',*,*,#8311,.T.);
#11828=ORIENTED_EDGE('',*,*,#8312,.T.);
#11829=ORIENTED_EDGE('',*,*,#8313,.T.);
#11830=ORIENTED_EDGE('',*,*,#8312,.F.);
#11831=ORIENTED_EDGE('',*,*,#8314,.T.);
#11832=ORIENTED_EDGE('',*,*,#8307,.F.);
#11833=ORIENTED_EDGE('',*,*,#8315,.T.);
#11834=ORIENTED_EDGE('',*,*,#8311,.F.);
#11835=ORIENTED_EDGE('',*,*,#8294,.F.);
#11836=ORIENTED_EDGE('',*,*,#8316,.T.);
#11837=ORIENTED_EDGE('',*,*,#8317,.F.);
#11838=ORIENTED_EDGE('',*,*,#8318,.F.);
#11839=ORIENTED_EDGE('',*,*,#8319,.T.);
#11840=ORIENTED_EDGE('',*,*,#8297,.F.);
#11841=ORIENTED_EDGE('',*,*,#8320,.T.);
#11842=ORIENTED_EDGE('',*,*,#8321,.F.);
#11843=ORIENTED_EDGE('',*,*,#8322,.F.);
#11844=ORIENTED_EDGE('',*,*,#8323,.F.);
#11845=ORIENTED_EDGE('',*,*,#8316,.F.);
#11846=ORIENTED_EDGE('',*,*,#8296,.F.);
#11847=ORIENTED_EDGE('',*,*,#8313,.F.);
#11848=ORIENTED_EDGE('',*,*,#8315,.F.);
#11849=ORIENTED_EDGE('',*,*,#8306,.F.);
#11850=ORIENTED_EDGE('',*,*,#8310,.F.);
#11851=ORIENTED_EDGE('',*,*,#8302,.F.);
#11852=ORIENTED_EDGE('',*,*,#8298,.F.);
#11853=ORIENTED_EDGE('',*,*,#8324,.T.);
#11854=ORIENTED_EDGE('',*,*,#8325,.F.);
#11855=ORIENTED_EDGE('',*,*,#8320,.F.);
#11856=ORIENTED_EDGE('',*,*,#8326,.T.);
#11857=ORIENTED_EDGE('',*,*,#8327,.F.);
#11858=ORIENTED_EDGE('',*,*,#8328,.T.);
#11859=ORIENTED_EDGE('',*,*,#8329,.T.);
#11860=ORIENTED_EDGE('',*,*,#8330,.T.);
#11861=ORIENTED_EDGE('',*,*,#8331,.F.);
#11862=ORIENTED_EDGE('',*,*,#8317,.T.);
#11863=ORIENTED_EDGE('',*,*,#8323,.T.);
#11864=ORIENTED_EDGE('',*,*,#8331,.T.);
#11865=ORIENTED_EDGE('',*,*,#8332,.T.);
#11866=ORIENTED_EDGE('',*,*,#8333,.T.);
#11867=ORIENTED_EDGE('',*,*,#8318,.T.);
#11868=ORIENTED_EDGE('',*,*,#8334,.T.);
#11869=ORIENTED_EDGE('',*,*,#8335,.T.);
#11870=ORIENTED_EDGE('',*,*,#8336,.T.);
#11871=ORIENTED_EDGE('',*,*,#8337,.T.);
#11872=ORIENTED_EDGE('',*,*,#8334,.F.);
#11873=ORIENTED_EDGE('',*,*,#8338,.T.);
#11874=ORIENTED_EDGE('',*,*,#8333,.F.);
#11875=ORIENTED_EDGE('',*,*,#8339,.T.);
#11876=ORIENTED_EDGE('',*,*,#8327,.T.);
#11877=ORIENTED_EDGE('',*,*,#8340,.T.);
#11878=ORIENTED_EDGE('',*,*,#8341,.T.);
#11879=ORIENTED_EDGE('',*,*,#8342,.T.);
#11880=ORIENTED_EDGE('',*,*,#8341,.F.);
#11881=ORIENTED_EDGE('',*,*,#8343,.T.);
#11882=ORIENTED_EDGE('',*,*,#8336,.F.);
#11883=ORIENTED_EDGE('',*,*,#8344,.T.);
#11884=ORIENTED_EDGE('',*,*,#8314,.F.);
#11885=ORIENTED_EDGE('',*,*,#8319,.F.);
#11886=ORIENTED_EDGE('',*,*,#8338,.F.);
#11887=ORIENTED_EDGE('',*,*,#8337,.F.);
#11888=ORIENTED_EDGE('',*,*,#8343,.F.);
#11889=ORIENTED_EDGE('',*,*,#8345,.F.);
#11890=ORIENTED_EDGE('',*,*,#8346,.F.);
#11891=ORIENTED_EDGE('',*,*,#8347,.F.);
#11892=ORIENTED_EDGE('',*,*,#8348,.F.);
#11893=ORIENTED_EDGE('',*,*,#8349,.F.);
#11894=ORIENTED_EDGE('',*,*,#8350,.F.);
#11895=ORIENTED_EDGE('',*,*,#8351,.F.);
#11896=ORIENTED_EDGE('',*,*,#8352,.F.);
#11897=ORIENTED_EDGE('',*,*,#8353,.F.);
#11898=ORIENTED_EDGE('',*,*,#8309,.F.);
#11899=ORIENTED_EDGE('',*,*,#8308,.F.);
#11900=ORIENTED_EDGE('',*,*,#8354,.F.);
#11901=ORIENTED_EDGE('',*,*,#8291,.F.);
#11902=ORIENTED_EDGE('',*,*,#8355,.F.);
#11903=ORIENTED_EDGE('',*,*,#8284,.F.);
#11904=ORIENTED_EDGE('',*,*,#8288,.T.);
#11905=ORIENTED_EDGE('',*,*,#8354,.T.);
#11906=ORIENTED_EDGE('',*,*,#8356,.T.);
#11907=ORIENTED_EDGE('',*,*,#8357,.T.);
#11908=ORIENTED_EDGE('',*,*,#8358,.T.);
#11909=ORIENTED_EDGE('',*,*,#8359,.T.);
#11910=ORIENTED_EDGE('',*,*,#8254,.T.);
#11911=ORIENTED_EDGE('',*,*,#8360,.T.);
#11912=ORIENTED_EDGE('',*,*,#8361,.T.);
#11913=ORIENTED_EDGE('',*,*,#8255,.T.);
#11914=ORIENTED_EDGE('',*,*,#8359,.F.);
#11915=ORIENTED_EDGE('',*,*,#8362,.T.);
#11916=ORIENTED_EDGE('',*,*,#8363,.T.);
#11917=ORIENTED_EDGE('',*,*,#8256,.T.);
#11918=ORIENTED_EDGE('',*,*,#8361,.F.);
#11919=ORIENTED_EDGE('',*,*,#8364,.T.);
#11920=ORIENTED_EDGE('',*,*,#8365,.T.);
#11921=ORIENTED_EDGE('',*,*,#8257,.T.);
#11922=ORIENTED_EDGE('',*,*,#8363,.F.);
#11923=ORIENTED_EDGE('',*,*,#8366,.T.);
#11924=ORIENTED_EDGE('',*,*,#8367,.T.);
#11925=ORIENTED_EDGE('',*,*,#8258,.T.);
#11926=ORIENTED_EDGE('',*,*,#8365,.F.);
#11927=ORIENTED_EDGE('',*,*,#8321,.T.);
#11928=ORIENTED_EDGE('',*,*,#8368,.T.);
#11929=ORIENTED_EDGE('',*,*,#8259,.T.);
#11930=ORIENTED_EDGE('',*,*,#8367,.F.);
#11931=ORIENTED_EDGE('',*,*,#8325,.T.);
#11932=ORIENTED_EDGE('',*,*,#8369,.T.);
#11933=ORIENTED_EDGE('',*,*,#8260,.T.);
#11934=ORIENTED_EDGE('',*,*,#8368,.F.);
#11935=ORIENTED_EDGE('',*,*,#8370,.T.);
#11936=ORIENTED_EDGE('',*,*,#8371,.T.);
#11937=ORIENTED_EDGE('',*,*,#8261,.T.);
#11938=ORIENTED_EDGE('',*,*,#8369,.F.);
#11939=ORIENTED_EDGE('',*,*,#8372,.T.);
#11940=ORIENTED_EDGE('',*,*,#8262,.T.);
#11941=ORIENTED_EDGE('',*,*,#8371,.F.);
#11942=ORIENTED_EDGE('',*,*,#8373,.T.);
#11943=ORIENTED_EDGE('',*,*,#8374,.T.);
#11944=ORIENTED_EDGE('',*,*,#8281,.F.);
#11945=ORIENTED_EDGE('',*,*,#8357,.F.);
#11946=ORIENTED_EDGE('',*,*,#8375,.T.);
#11947=ORIENTED_EDGE('',*,*,#8360,.F.);
#11948=ORIENTED_EDGE('',*,*,#8376,.T.);
#11949=ORIENTED_EDGE('',*,*,#8377,.T.);
#11950=ORIENTED_EDGE('',*,*,#8355,.T.);
#11951=ORIENTED_EDGE('',*,*,#8378,.T.);
#11952=ORIENTED_EDGE('',*,*,#8374,.F.);
#11953=ORIENTED_EDGE('',*,*,#8330,.F.);
#11954=ORIENTED_EDGE('',*,*,#8322,.T.);
#11955=ORIENTED_EDGE('',*,*,#8366,.F.);
#11956=ORIENTED_EDGE('',*,*,#8379,.F.);
#11957=ORIENTED_EDGE('',*,*,#8328,.F.);
#11958=ORIENTED_EDGE('',*,*,#8342,.F.);
#11959=ORIENTED_EDGE('',*,*,#8344,.F.);
#11960=ORIENTED_EDGE('',*,*,#8335,.F.);
#11961=ORIENTED_EDGE('',*,*,#8339,.F.);
#11962=ORIENTED_EDGE('',*,*,#8332,.F.);
#11963=ORIENTED_EDGE('',*,*,#8329,.F.);
#11964=ORIENTED_EDGE('',*,*,#8379,.T.);
#11965=ORIENTED_EDGE('',*,*,#8364,.F.);
#11966=ORIENTED_EDGE('',*,*,#8380,.F.);
#11967=ORIENTED_EDGE('',*,*,#8381,.F.);
#11968=ORIENTED_EDGE('',*,*,#8382,.F.);
#11969=ORIENTED_EDGE('',*,*,#8362,.F.);
#11970=ORIENTED_EDGE('',*,*,#8383,.F.);
#11971=ORIENTED_EDGE('',*,*,#8384,.F.);
#11972=ORIENTED_EDGE('',*,*,#8385,.F.);
#11973=ORIENTED_EDGE('',*,*,#8386,.F.);
#11974=ORIENTED_EDGE('',*,*,#8387,.F.);
#11975=ORIENTED_EDGE('',*,*,#8388,.F.);
#11976=ORIENTED_EDGE('',*,*,#8389,.F.);
#11977=ORIENTED_EDGE('',*,*,#8390,.F.);
#11978=ORIENTED_EDGE('',*,*,#8380,.T.);
#11979=ORIENTED_EDGE('',*,*,#8293,.F.);
#11980=ORIENTED_EDGE('',*,*,#8263,.F.);
#11981=ORIENTED_EDGE('',*,*,#8378,.F.);
#11982=ORIENTED_EDGE('',*,*,#8290,.F.);
#11983=ORIENTED_EDGE('',*,*,#8282,.F.);
#11984=ORIENTED_EDGE('',*,*,#8376,.F.);
#11985=ORIENTED_EDGE('',*,*,#8253,.F.);
#11986=ORIENTED_EDGE('',*,*,#8286,.F.);
#11987=ORIENTED_EDGE('',*,*,#8391,.T.);
#11988=ORIENTED_EDGE('',*,*,#8392,.F.);
#11989=ORIENTED_EDGE('',*,*,#8393,.T.);
#11990=ORIENTED_EDGE('',*,*,#8394,.T.);
#11991=ORIENTED_EDGE('',*,*,#8395,.T.);
#11992=ORIENTED_EDGE('',*,*,#8396,.F.);
#11993=ORIENTED_EDGE('',*,*,#8397,.T.);
#11994=ORIENTED_EDGE('',*,*,#8398,.T.);
#11995=ORIENTED_EDGE('',*,*,#8396,.T.);
#11996=ORIENTED_EDGE('',*,*,#8399,.T.);
#11997=ORIENTED_EDGE('',*,*,#8400,.T.);
#11998=ORIENTED_EDGE('',*,*,#8401,.T.);
#11999=ORIENTED_EDGE('',*,*,#8402,.T.);
#12000=ORIENTED_EDGE('',*,*,#8403,.T.);
#12001=ORIENTED_EDGE('',*,*,#8404,.T.);
#12002=ORIENTED_EDGE('',*,*,#8351,.T.);
#12003=ORIENTED_EDGE('',*,*,#8402,.F.);
#12004=ORIENTED_EDGE('',*,*,#8350,.T.);
#12005=ORIENTED_EDGE('',*,*,#8400,.F.);
#12006=ORIENTED_EDGE('',*,*,#8405,.T.);
#12007=ORIENTED_EDGE('',*,*,#8392,.T.);
#12008=ORIENTED_EDGE('',*,*,#8406,.T.);
#12009=ORIENTED_EDGE('',*,*,#8407,.T.);
#12010=ORIENTED_EDGE('',*,*,#8408,.T.);
#12011=ORIENTED_EDGE('',*,*,#8407,.F.);
#12012=ORIENTED_EDGE('',*,*,#8352,.T.);
#12013=ORIENTED_EDGE('',*,*,#8404,.F.);
#12014=ORIENTED_EDGE('',*,*,#8409,.T.);
#12015=ORIENTED_EDGE('',*,*,#8304,.F.);
#12016=ORIENTED_EDGE('',*,*,#8353,.T.);
#12017=ORIENTED_EDGE('',*,*,#8406,.F.);
#12018=ORIENTED_EDGE('',*,*,#8391,.F.);
#12019=ORIENTED_EDGE('',*,*,#8410,.T.);
#12020=ORIENTED_EDGE('',*,*,#8300,.F.);
#12021=ORIENTED_EDGE('',*,*,#8301,.F.);
#12022=ORIENTED_EDGE('',*,*,#8410,.F.);
#12023=ORIENTED_EDGE('',*,*,#8394,.F.);
#12024=ORIENTED_EDGE('',*,*,#8411,.T.);
#12025=ORIENTED_EDGE('',*,*,#8370,.F.);
#12026=ORIENTED_EDGE('',*,*,#8324,.F.);
#12027=ORIENTED_EDGE('',*,*,#8372,.F.);
#12028=ORIENTED_EDGE('',*,*,#8411,.F.);
#12029=ORIENTED_EDGE('',*,*,#8393,.F.);
#12030=ORIENTED_EDGE('',*,*,#8408,.F.);
#12031=ORIENTED_EDGE('',*,*,#8409,.F.);
#12032=ORIENTED_EDGE('',*,*,#8403,.F.);
#12033=ORIENTED_EDGE('',*,*,#8405,.F.);
#12034=ORIENTED_EDGE('',*,*,#8399,.F.);
#12035=ORIENTED_EDGE('',*,*,#8395,.F.);
#12036=ORIENTED_EDGE('',*,*,#8412,.T.);
#12037=ORIENTED_EDGE('',*,*,#8413,.T.);
#12038=ORIENTED_EDGE('',*,*,#8414,.F.);
#12039=ORIENTED_EDGE('',*,*,#8384,.T.);
#12040=ORIENTED_EDGE('',*,*,#8415,.T.);
#12041=ORIENTED_EDGE('',*,*,#8390,.T.);
#12042=ORIENTED_EDGE('',*,*,#8416,.F.);
#12043=ORIENTED_EDGE('',*,*,#8417,.T.);
#12044=ORIENTED_EDGE('',*,*,#8381,.T.);
#12045=ORIENTED_EDGE('',*,*,#8416,.T.);
#12046=ORIENTED_EDGE('',*,*,#8389,.T.);
#12047=ORIENTED_EDGE('',*,*,#8418,.T.);
#12048=ORIENTED_EDGE('',*,*,#8419,.T.);
#12049=ORIENTED_EDGE('',*,*,#8420,.T.);
#12050=ORIENTED_EDGE('',*,*,#8387,.T.);
#12051=ORIENTED_EDGE('',*,*,#8421,.T.);
#12052=ORIENTED_EDGE('',*,*,#8347,.T.);
#12053=ORIENTED_EDGE('',*,*,#8420,.F.);
#12054=ORIENTED_EDGE('',*,*,#8346,.T.);
#12055=ORIENTED_EDGE('',*,*,#8418,.F.);
#12056=ORIENTED_EDGE('',*,*,#8388,.T.);
#12057=ORIENTED_EDGE('',*,*,#8414,.T.);
#12058=ORIENTED_EDGE('',*,*,#8422,.T.);
#12059=ORIENTED_EDGE('',*,*,#8423,.T.);
#12060=ORIENTED_EDGE('',*,*,#8385,.T.);
#12061=ORIENTED_EDGE('',*,*,#8423,.F.);
#12062=ORIENTED_EDGE('',*,*,#8348,.T.);
#12063=ORIENTED_EDGE('',*,*,#8421,.F.);
#12064=ORIENTED_EDGE('',*,*,#8386,.T.);
#12065=ORIENTED_EDGE('',*,*,#8326,.F.);
#12066=ORIENTED_EDGE('',*,*,#8382,.T.);
#12067=ORIENTED_EDGE('',*,*,#8417,.F.);
#12068=ORIENTED_EDGE('',*,*,#8419,.F.);
#12069=ORIENTED_EDGE('',*,*,#8345,.T.);
#12070=ORIENTED_EDGE('',*,*,#8340,.F.);
#12071=ORIENTED_EDGE('',*,*,#8401,.F.);
#12072=ORIENTED_EDGE('',*,*,#8349,.T.);
#12073=ORIENTED_EDGE('',*,*,#8422,.F.);
#12074=ORIENTED_EDGE('',*,*,#8413,.F.);
#12075=ORIENTED_EDGE('',*,*,#8424,.T.);
#12076=ORIENTED_EDGE('',*,*,#8397,.F.);
#12077=ORIENTED_EDGE('',*,*,#8373,.F.);
#12078=ORIENTED_EDGE('',*,*,#8412,.F.);
#12079=ORIENTED_EDGE('',*,*,#8398,.F.);
#12080=ORIENTED_EDGE('',*,*,#8424,.F.);
#12081=ORIENTED_EDGE('',*,*,#8415,.F.);
#12082=ORIENTED_EDGE('',*,*,#8383,.T.);
#12083=ORIENTED_EDGE('',*,*,#8358,.F.);
#12084=ORIENTED_EDGE('',*,*,#8375,.F.);
#12085=ORIENTED_EDGE('',*,*,#8356,.F.);
#12086=ORIENTED_EDGE('',*,*,#8377,.F.);
#12087=ORIENTED_EDGE('',*,*,#8251,.F.);
#12088=ORIENTED_EDGE('',*,*,#8425,.T.);
#12089=ORIENTED_EDGE('',*,*,#8426,.T.);
#12090=ORIENTED_EDGE('',*,*,#8272,.F.);
#12091=ORIENTED_EDGE('',*,*,#8249,.F.);
#12092=ORIENTED_EDGE('',*,*,#8427,.T.);
#12093=ORIENTED_EDGE('',*,*,#8428,.T.);
#12094=ORIENTED_EDGE('',*,*,#8425,.F.);
#12095=ORIENTED_EDGE('',*,*,#8246,.F.);
#12096=ORIENTED_EDGE('',*,*,#8429,.T.);
#12097=ORIENTED_EDGE('',*,*,#8430,.T.);
#12098=ORIENTED_EDGE('',*,*,#8427,.F.);
#12099=ORIENTED_EDGE('',*,*,#8243,.F.);
#12100=ORIENTED_EDGE('',*,*,#8267,.T.);
#12101=ORIENTED_EDGE('',*,*,#8431,.T.);
#12102=ORIENTED_EDGE('',*,*,#8429,.F.);
#12103=ORIENTED_EDGE('',*,*,#8271,.F.);
#12104=ORIENTED_EDGE('',*,*,#8273,.F.);
#12105=ORIENTED_EDGE('',*,*,#8426,.F.);
#12106=ORIENTED_EDGE('',*,*,#8428,.F.);
#12107=ORIENTED_EDGE('',*,*,#8430,.F.);
#12108=ORIENTED_EDGE('',*,*,#8431,.F.);
#12109=ORIENTED_EDGE('',*,*,#8266,.F.);
#12110=ORIENTED_EDGE('',*,*,#8269,.F.);
#12881=PLANE('',#14803);
#12882=PLANE('',#14807);
#12883=PLANE('',#14811);
#12884=PLANE('',#14815);
#12885=PLANE('',#14819);
#12886=PLANE('',#14826);
#12887=PLANE('',#14829);
#12888=PLANE('',#14830);
#12889=PLANE('',#14831);
#12890=PLANE('',#14832);
#12891=PLANE('',#14833);
#12892=PLANE('',#14834);
#12893=PLANE('',#14835);
#12894=PLANE('',#14836);
#12895=PLANE('',#14837);
#12896=PLANE('',#14842);
#12897=PLANE('',#14848);
#12898=PLANE('',#14851);
#12899=PLANE('',#14852);
#12900=PLANE('',#14853);
#12901=PLANE('',#14856);
#12902=PLANE('',#14859);
#12903=PLANE('',#14861);
#12904=PLANE('',#14864);
#12905=PLANE('',#14865);
#12906=PLANE('',#14866);
#12907=PLANE('',#14868);
#12908=PLANE('',#14871);
#12909=PLANE('',#14872);
#12910=PLANE('',#14876);
#12911=PLANE('',#14881);
#12912=PLANE('',#14884);
#12913=PLANE('',#14887);
#12914=PLANE('',#14888);
#13629=ADVANCED_FACE('',(#1866),#12881,.T.);
#13630=ADVANCED_FACE('',(#1867),#1228,.F.);
#13631=ADVANCED_FACE('',(#1868),#12882,.T.);
#13632=ADVANCED_FACE('',(#1869),#1229,.F.);
#13633=ADVANCED_FACE('',(#1870),#12883,.T.);
#13634=ADVANCED_FACE('',(#1871),#1230,.F.);
#13635=ADVANCED_FACE('',(#1872),#12884,.T.);
#13636=ADVANCED_FACE('',(#1873),#1231,.F.);
#13637=ADVANCED_FACE('',(#1874),#12885,.T.);
#13638=ADVANCED_FACE('',(#1875),#760,.F.);
#13639=ADVANCED_FACE('',(#1876),#12886,.F.);
#13640=ADVANCED_FACE('',(#1877),#761,.F.);
#13641=ADVANCED_FACE('',(#1878),#12887,.F.);
#13642=ADVANCED_FACE('',(#1879),#12888,.T.);
#13643=ADVANCED_FACE('',(#1880),#12889,.T.);
#13644=ADVANCED_FACE('',(#1881),#12890,.T.);
#13645=ADVANCED_FACE('',(#1882),#12891,.T.);
#13646=ADVANCED_FACE('',(#1883),#12892,.T.);
#13647=ADVANCED_FACE('',(#1884),#12893,.T.);
#13648=ADVANCED_FACE('',(#1885),#12894,.T.);
#13649=ADVANCED_FACE('',(#1886),#12895,.T.);
#13650=ADVANCED_FACE('',(#1887),#511,.T.);
#13651=ADVANCED_FACE('',(#1888),#512,.T.);
#13652=ADVANCED_FACE('',(#1889),#513,.T.);
#13653=ADVANCED_FACE('',(#1890),#1232,.T.);
#13654=ADVANCED_FACE('',(#1891),#514,.T.);
#13655=ADVANCED_FACE('',(#1892),#515,.T.);
#13656=ADVANCED_FACE('',(#1893),#516,.T.);
#13657=ADVANCED_FACE('',(#1894),#762,.T.);
#13658=ADVANCED_FACE('',(#1895),#12896,.T.);
#13659=ADVANCED_FACE('',(#1896),#763,.T.);
#13660=ADVANCED_FACE('',(#1897),#517,.T.);
#13661=ADVANCED_FACE('',(#1898),#518,.T.);
#13662=ADVANCED_FACE('',(#1899),#519,.T.);
#13663=ADVANCED_FACE('',(#1900),#1233,.T.);
#13664=ADVANCED_FACE('',(#1901),#520,.T.);
#13665=ADVANCED_FACE('',(#1902),#521,.T.);
#13666=ADVANCED_FACE('',(#1903),#522,.T.);
#13667=ADVANCED_FACE('',(#1904),#12897,.F.);
#13668=ADVANCED_FACE('',(#1905),#12898,.T.);
#13669=ADVANCED_FACE('',(#1906),#12899,.T.);
#13670=ADVANCED_FACE('',(#1907),#12900,.T.);
#13671=ADVANCED_FACE('',(#1908),#1234,.T.);
#13672=ADVANCED_FACE('',(#1909),#12901,.T.);
#13673=ADVANCED_FACE('',(#1910),#1235,.T.);
#13674=ADVANCED_FACE('',(#1911),#12902,.T.);
#13675=ADVANCED_FACE('',(#1912),#1236,.T.);
#13676=ADVANCED_FACE('',(#1913),#12903,.T.);
#13677=ADVANCED_FACE('',(#1914),#1237,.T.);
#13678=ADVANCED_FACE('',(#1915),#12904,.T.);
#13679=ADVANCED_FACE('',(#1916),#12905,.T.);
#13680=ADVANCED_FACE('',(#1917),#12906,.T.);
#13681=ADVANCED_FACE('',(#1918),#764,.T.);
#13682=ADVANCED_FACE('',(#1919),#12907,.T.);
#13683=ADVANCED_FACE('',(#1920),#765,.T.);
#13684=ADVANCED_FACE('',(#1921),#12908,.T.);
#13685=ADVANCED_FACE('',(#1922),#12909,.T.);
#13686=ADVANCED_FACE('',(#1923),#523,.T.);
#13687=ADVANCED_FACE('',(#1924),#524,.T.);
#13688=ADVANCED_FACE('',(#1925),#525,.T.);
#13689=ADVANCED_FACE('',(#1926),#1238,.T.);
#13690=ADVANCED_FACE('',(#1927),#526,.T.);
#13691=ADVANCED_FACE('',(#1928),#527,.T.);
#13692=ADVANCED_FACE('',(#1929),#528,.T.);
#13693=ADVANCED_FACE('',(#1930),#766,.T.);
#13694=ADVANCED_FACE('',(#1931),#12910,.T.);
#13695=ADVANCED_FACE('',(#1932),#767,.T.);
#13696=ADVANCED_FACE('',(#1933),#529,.T.);
#13697=ADVANCED_FACE('',(#1934),#530,.T.);
#13698=ADVANCED_FACE('',(#1935),#531,.T.);
#13699=ADVANCED_FACE('',(#1936),#1239,.T.);
#13700=ADVANCED_FACE('',(#1937),#532,.T.);
#13701=ADVANCED_FACE('',(#1938),#533,.T.);
#13702=ADVANCED_FACE('',(#1939),#534,.T.);
#13703=ADVANCED_FACE('',(#1940),#768,.T.);
#13704=ADVANCED_FACE('',(#1941),#769,.T.);
#13705=ADVANCED_FACE('',(#1942),#12911,.T.);
#13706=ADVANCED_FACE('',(#1943),#770,.F.);
#13707=ADVANCED_FACE('',(#1944),#12912,.F.);
#13708=ADVANCED_FACE('',(#1945),#771,.F.);
#13709=ADVANCED_FACE('',(#1946),#12913,.F.);
#13710=ADVANCED_FACE('',(#1947),#12914,.T.);
#13816=CLOSED_SHELL('',(#13629,#13630,#13631,#13632,#13633,#13634,#13635,
#13636,#13637,#13638,#13639,#13640,#13641,#13642,#13643,#13644,#13645,#13646,
#13647,#13648,#13649,#13650,#13651,#13652,#13653,#13654,#13655,#13656,#13657,
#13658,#13659,#13660,#13661,#13662,#13663,#13664,#13665,#13666,#13667,#13668,
#13669,#13670,#13671,#13672,#13673,#13674,#13675,#13676,#13677,#13678,#13679,
#13680,#13681,#13682,#13683,#13684,#13685,#13686,#13687,#13688,#13689,#13690,
#13691,#13692,#13693,#13694,#13695,#13696,#13697,#13698,#13699,#13700,#13701,
#13702,#13703,#13704,#13705,#13706,#13707,#13708,#13709,#13710));
#14802=AXIS2_PLACEMENT_3D('',#29366,#17608,#17609);
#14803=AXIS2_PLACEMENT_3D('',#29367,#17610,#17611);
#14804=AXIS2_PLACEMENT_3D('',#29380,#17618,#17619);
#14805=AXIS2_PLACEMENT_3D('',#29384,#17621,#17622);
#14806=AXIS2_PLACEMENT_3D('',#29385,#17623,#17624);
#14807=AXIS2_PLACEMENT_3D('',#29386,#17625,#17626);
#14808=AXIS2_PLACEMENT_3D('',#29392,#17630,#17631);
#14809=AXIS2_PLACEMENT_3D('',#29396,#17633,#17634);
#14810=AXIS2_PLACEMENT_3D('',#29397,#17635,#17636);
#14811=AXIS2_PLACEMENT_3D('',#29398,#17637,#17638);
#14812=AXIS2_PLACEMENT_3D('',#29404,#17642,#17643);
#14813=AXIS2_PLACEMENT_3D('',#29408,#17645,#17646);
#14814=AXIS2_PLACEMENT_3D('',#29409,#17647,#17648);
#14815=AXIS2_PLACEMENT_3D('',#29410,#17649,#17650);
#14816=AXIS2_PLACEMENT_3D('',#29416,#17654,#17655);
#14817=AXIS2_PLACEMENT_3D('',#29417,#17656,#17657);
#14818=AXIS2_PLACEMENT_3D('',#29418,#17658,#17659);
#14819=AXIS2_PLACEMENT_3D('',#29419,#17660,#17661);
#14820=AXIS2_PLACEMENT_3D('',#29427,#17665,#17666);
#14821=AXIS2_PLACEMENT_3D('',#29431,#17668,#17669);
#14822=AXIS2_PLACEMENT_3D('',#29435,#17671,#17672);
#14823=AXIS2_PLACEMENT_3D('',#29439,#17674,#17675);
#14824=AXIS2_PLACEMENT_3D('',#29445,#17679,#17680);
#14825=AXIS2_PLACEMENT_3D('',#29449,#17682,#17683);
#14826=AXIS2_PLACEMENT_3D('',#29451,#17685,#17686);
#14827=AXIS2_PLACEMENT_3D('',#29455,#17689,#17690);
#14828=AXIS2_PLACEMENT_3D('',#29458,#17692,#17693);
#14829=AXIS2_PLACEMENT_3D('',#29459,#17694,#17695);
#14830=AXIS2_PLACEMENT_3D('',#29463,#17698,#17699);
#14831=AXIS2_PLACEMENT_3D('',#29470,#17703,#17704);
#14832=AXIS2_PLACEMENT_3D('',#29478,#17709,#17710);
#14833=AXIS2_PLACEMENT_3D('',#29486,#17715,#17716);
#14834=AXIS2_PLACEMENT_3D('',#29489,#17719,#17720);
#14835=AXIS2_PLACEMENT_3D('',#29493,#17723,#17724);
#14836=AXIS2_PLACEMENT_3D('',#29499,#17728,#17729);
#14837=AXIS2_PLACEMENT_3D('',#29502,#17732,#17733);
#14838=AXIS2_PLACEMENT_3D('',#29946,#17737,#17738);
#14839=AXIS2_PLACEMENT_3D('',#29951,#17740,#17741);
#14840=AXIS2_PLACEMENT_3D('',#29954,#17743,#17744);
#14841=AXIS2_PLACEMENT_3D('',#30036,#17746,#17747);
#14842=AXIS2_PLACEMENT_3D('',#30141,#17750,#17751);
#14843=AXIS2_PLACEMENT_3D('',#30149,#17756,#17757);
#14844=AXIS2_PLACEMENT_3D('',#30152,#17759,#17760);
#14845=AXIS2_PLACEMENT_3D('',#30500,#17763,#17764);
#14846=AXIS2_PLACEMENT_3D('',#30505,#17766,#17767);
#14847=AXIS2_PLACEMENT_3D('',#30508,#17769,#17770);
#14848=AXIS2_PLACEMENT_3D('',#30590,#17772,#17773);
#14849=AXIS2_PLACEMENT_3D('',#30599,#17775,#17776);
#14850=AXIS2_PLACEMENT_3D('',#30613,#17778,#17779);
#14851=AXIS2_PLACEMENT_3D('',#30620,#17781,#17782);
#14852=AXIS2_PLACEMENT_3D('',#30624,#17785,#17786);
#14853=AXIS2_PLACEMENT_3D('',#30628,#17789,#17790);
#14854=AXIS2_PLACEMENT_3D('',#30634,#17794,#17795);
#14855=AXIS2_PLACEMENT_3D('',#30637,#17797,#17798);
#14856=AXIS2_PLACEMENT_3D('',#30638,#17799,#17800);
#14857=AXIS2_PLACEMENT_3D('',#30642,#17803,#17804);
#14858=AXIS2_PLACEMENT_3D('',#30644,#17806,#17807);
#14859=AXIS2_PLACEMENT_3D('',#30645,#17808,#17809);
#14860=AXIS2_PLACEMENT_3D('',#30647,#17811,#17812);
#14861=AXIS2_PLACEMENT_3D('',#30649,#17814,#17815);
#14862=AXIS2_PLACEMENT_3D('',#30653,#17818,#17819);
#14863=AXIS2_PLACEMENT_3D('',#30656,#17821,#17822);
#14864=AXIS2_PLACEMENT_3D('',#30657,#17823,#17824);
#14865=AXIS2_PLACEMENT_3D('',#30661,#17827,#17828);
#14866=AXIS2_PLACEMENT_3D('',#30664,#17831,#17832);
#14867=AXIS2_PLACEMENT_3D('',#30667,#17835,#17836);
#14868=AXIS2_PLACEMENT_3D('',#30669,#17838,#17839);
#14869=AXIS2_PLACEMENT_3D('',#30675,#17843,#17844);
#14870=AXIS2_PLACEMENT_3D('',#30761,#17846,#17847);
#14871=AXIS2_PLACEMENT_3D('',#30850,#17848,#17849);
#14872=AXIS2_PLACEMENT_3D('',#30851,#17850,#17851);
#14873=AXIS2_PLACEMENT_3D('',#31302,#17855,#17856);
#14874=AXIS2_PLACEMENT_3D('',#31306,#17858,#17859);
#14875=AXIS2_PLACEMENT_3D('',#31380,#17862,#17863);
#14876=AXIS2_PLACEMENT_3D('',#31382,#17865,#17866);
#14877=AXIS2_PLACEMENT_3D('',#31384,#17868,#17869);
#14878=AXIS2_PLACEMENT_3D('',#31684,#17873,#17874);
#14879=AXIS2_PLACEMENT_3D('',#31745,#17878,#17879);
#14880=AXIS2_PLACEMENT_3D('',#31746,#17880,#17881);
#14881=AXIS2_PLACEMENT_3D('',#31748,#17883,#17884);
#14882=AXIS2_PLACEMENT_3D('',#31749,#17885,#17886);
#14883=AXIS2_PLACEMENT_3D('',#31752,#17888,#17889);
#14884=AXIS2_PLACEMENT_3D('',#31753,#17890,#17891);
#14885=AXIS2_PLACEMENT_3D('',#31757,#17894,#17895);
#14886=AXIS2_PLACEMENT_3D('',#31760,#17897,#17898);
#14887=AXIS2_PLACEMENT_3D('',#31761,#17899,#17900);
#14888=AXIS2_PLACEMENT_3D('',#31763,#17902,#17903);
#17608=DIRECTION('axis',(0.,0.,1.));
#17609=DIRECTION('refdir',(1.,0.,0.));
#17610=DIRECTION('center_axis',(0.,0.707106781186548,0.707106781186548));
#17611=DIRECTION('ref_axis',(1.,0.,0.));
#17612=DIRECTION('',(0.,-0.707106781186548,0.707106781186548));
#17613=DIRECTION('',(1.,0.,0.));
#17614=DIRECTION('',(1.,0.,0.));
#17615=DIRECTION('',(1.,0.,0.));
#17616=DIRECTION('',(0.,0.707106781186548,-0.707106781186548));
#17617=DIRECTION('',(-1.,0.,0.));
#17618=DIRECTION('center_axis',(0.,0.,1.));
#17619=DIRECTION('ref_axis',(-1.,-1.97372982155583E-15,0.));
#17620=DIRECTION('',(-0.707106781186549,0.,0.707106781186546));
#17621=DIRECTION('center_axis',(0.,0.,1.));
#17622=DIRECTION('ref_axis',(-1.,-1.97372982155583E-15,0.));
#17623=DIRECTION('center_axis',(0.,0.,-1.));
#17624=DIRECTION('ref_axis',(-1.,-1.97372982155583E-15,0.));
#17625=DIRECTION('center_axis',(0.707106781186549,0.,0.707106781186546));
#17626=DIRECTION('ref_axis',(0.707106781186546,0.,-0.707106781186549));
#17627=DIRECTION('',(-0.707106781186546,0.,0.707106781186549));
#17628=DIRECTION('',(0.,-1.,0.));
#17629=DIRECTION('',(0.,1.,0.));
#17630=DIRECTION('center_axis',(0.,0.,1.));
#17631=DIRECTION('ref_axis',(-2.46716227694479E-15,1.,0.));
#17632=DIRECTION('',(-1.57009245868378E-15,0.707106781186548,0.707106781186548));
#17633=DIRECTION('center_axis',(0.,0.,1.));
#17634=DIRECTION('ref_axis',(-2.46716227694479E-15,1.,0.));
#17635=DIRECTION('center_axis',(0.,0.,-1.));
#17636=DIRECTION('ref_axis',(-2.46716227694479E-15,1.,0.));
#17637=DIRECTION('center_axis',(0.,-0.707106781186551,0.707106781186544));
#17638=DIRECTION('ref_axis',(1.,0.,0.));
#17639=DIRECTION('',(0.,0.707106781186544,0.707106781186551));
#17640=DIRECTION('',(-1.,0.,0.));
#17641=DIRECTION('',(1.,0.,0.));
#17642=DIRECTION('center_axis',(0.,0.,1.));
#17643=DIRECTION('ref_axis',(1.,3.94745964311165E-15,0.));
#17644=DIRECTION('',(0.707106781186548,0.,0.707106781186548));
#17645=DIRECTION('center_axis',(0.,0.,1.));
#17646=DIRECTION('ref_axis',(1.,3.94745964311165E-15,0.));
#17647=DIRECTION('center_axis',(0.,0.,-1.));
#17648=DIRECTION('ref_axis',(1.,3.94745964311165E-15,0.));
#17649=DIRECTION('center_axis',(-0.707106781186548,0.,0.707106781186548));
#17650=DIRECTION('ref_axis',(0.707106781186548,0.,0.707106781186548));
#17651=DIRECTION('',(0.707106781186548,0.,0.707106781186548));
#17652=DIRECTION('',(0.,1.,0.));
#17653=DIRECTION('',(0.,-1.,0.));
#17654=DIRECTION('center_axis',(0.,0.,1.));
#17655=DIRECTION('ref_axis',(9.86864910777915E-16,-1.,0.));
#17656=DIRECTION('center_axis',(0.,0.,1.));
#17657=DIRECTION('ref_axis',(9.86864910777915E-16,-1.,0.));
#17658=DIRECTION('center_axis',(0.,0.,-1.));
#17659=DIRECTION('ref_axis',(9.86864910777915E-16,-1.,0.));
#17660=DIRECTION('center_axis',(0.,0.,1.));
#17661=DIRECTION('ref_axis',(1.,0.,0.));
#17662=DIRECTION('',(0.707106781186541,-0.707106781186554,0.));
#17663=DIRECTION('',(0.,-1.,0.));
#17664=DIRECTION('',(-1.,0.,0.));
#17665=DIRECTION('center_axis',(0.,0.,-1.));
#17666=DIRECTION('ref_axis',(1.26882631385732E-15,-1.,0.));
#17667=DIRECTION('',(0.,-1.,0.));
#17668=DIRECTION('center_axis',(0.,0.,-1.));
#17669=DIRECTION('ref_axis',(1.,1.26882631385732E-15,0.));
#17670=DIRECTION('',(1.,0.,0.));
#17671=DIRECTION('center_axis',(0.,0.,-1.));
#17672=DIRECTION('ref_axis',(-9.51619735392991E-16,1.,0.));
#17673=DIRECTION('',(0.,1.,0.));
#17674=DIRECTION('center_axis',(0.,0.,-1.));
#17675=DIRECTION('ref_axis',(-1.,-1.26882631385732E-15,0.));
#17676=DIRECTION('',(-1.,0.,0.));
#17677=DIRECTION('',(0.,1.,0.));
#17678=DIRECTION('',(0.707106781186543,0.707106781186552,0.));
#17679=DIRECTION('center_axis',(0.,0.,-1.));
#17680=DIRECTION('ref_axis',(-2.46716227694479E-15,1.,0.));
#17681=DIRECTION('',(0.,0.,-1.));
#17682=DIRECTION('center_axis',(0.,0.,-1.));
#17683=DIRECTION('ref_axis',(-2.46716227694479E-15,1.,0.));
#17684=DIRECTION('',(0.,0.,-1.));
#17685=DIRECTION('center_axis',(-1.,0.,0.));
#17686=DIRECTION('ref_axis',(0.,1.,0.));
#17687=DIRECTION('',(0.,0.,-1.));
#17688=DIRECTION('',(0.,1.,0.));
#17689=DIRECTION('center_axis',(0.,0.,-1.));
#17690=DIRECTION('ref_axis',(-1.,-1.97372982155583E-15,0.));
#17691=DIRECTION('',(0.,0.,-1.));
#17692=DIRECTION('center_axis',(0.,0.,-1.));
#17693=DIRECTION('ref_axis',(-1.,-1.97372982155583E-15,0.));
#17694=DIRECTION('center_axis',(0.,-1.,0.));
#17695=DIRECTION('ref_axis',(-1.,0.,0.));
#17696=DIRECTION('',(0.,0.,-1.));
#17697=DIRECTION('',(-1.,0.,0.));
#17698=DIRECTION('center_axis',(0.57735026918963,0.57735026918962,0.577350269189628));
#17699=DIRECTION('ref_axis',(0.707106781186546,0.,-0.707106781186549));
#17700=DIRECTION('',(0.707106781186541,-0.707106781186554,0.));
#17701=DIRECTION('',(0.,0.707106781186552,-0.707106781186543));
#17702=DIRECTION('',(-0.707106781186546,0.,0.707106781186549));
#17703=DIRECTION('center_axis',(0.,0.707106781186543,0.707106781186552));
#17704=DIRECTION('ref_axis',(1.,0.,0.));
#17705=DIRECTION('',(0.577350269189623,-0.577350269189631,0.577350269189623));
#17706=DIRECTION('',(1.,0.,0.));
#17707=DIRECTION('',(-1.,0.,0.));
#17708=DIRECTION('',(-0.577350269189623,-0.577350269189631,0.577350269189623));
#17709=DIRECTION('center_axis',(0.707106781186549,0.,0.707106781186546));
#17710=DIRECTION('ref_axis',(0.707106781186546,0.,-0.707106781186549));
#17711=DIRECTION('',(0.577350269189628,0.577350269189618,-0.577350269189631));
#17712=DIRECTION('',(0.,1.,0.));
#17713=DIRECTION('',(0.,-1.,0.));
#17714=DIRECTION('',(0.577350269189628,-0.577350269189618,-0.577350269189631));
#17715=DIRECTION('center_axis',(0.707106781186554,0.707106781186541,0.));
#17716=DIRECTION('ref_axis',(0.,0.,-1.));
#17717=DIRECTION('',(0.,0.,1.));
#17718=DIRECTION('',(0.,0.,-1.));
#17719=DIRECTION('center_axis',(0.,0.,1.));
#17720=DIRECTION('ref_axis',(-1.,0.,0.));
#17721=DIRECTION('',(0.,1.,0.));
#17722=DIRECTION('',(-1.,0.,0.));
#17723=DIRECTION('center_axis',(-0.707106781186548,0.,0.707106781186548));
#17724=DIRECTION('ref_axis',(0.707106781186548,0.,0.707106781186548));
#17725=DIRECTION('',(0.577350269189623,0.577350269189631,0.577350269189623));
#17726=DIRECTION('',(0.,-1.,0.));
#17727=DIRECTION('',(0.707106781186547,0.,0.707106781186547));
#17728=DIRECTION('center_axis',(-0.707106781186552,0.707106781186543,0.));
#17729=DIRECTION('ref_axis',(0.,0.,1.));
#17730=DIRECTION('',(0.,0.,-1.));
#17731=DIRECTION('',(0.,0.,1.));
#17732=DIRECTION('center_axis',(0.,1.,0.));
#17733=DIRECTION('ref_axis',(1.,0.,0.));
#17734=DIRECTION('',(0.881917103688204,0.,-0.471404520791018));
#17735=DIRECTION('',(0.,0.881917103688206,0.471404520791014));
#17736=DIRECTION('',(0.465319173178999,-0.504527148397124,-0.727276029855432));
#17737=DIRECTION('center_axis',(0.,0.,1.));
#17738=DIRECTION('ref_axis',(-9.5161973539299E-16,1.,0.));
#17739=DIRECTION('',(-0.5050762722761,0.494871659305393,0.707106781186552));
#17740=DIRECTION('center_axis',(0.,0.,-1.));
#17741=DIRECTION('ref_axis',(-9.51619735392991E-16,1.,0.));
#17742=DIRECTION('',(0.49487165930539,-0.505076272276101,-0.707106781186553));
#17743=DIRECTION('center_axis',(0.,0.,1.));
#17744=DIRECTION('ref_axis',(-9.51619735392991E-16,1.,0.));
#17745=DIRECTION('',(-0.504527148397126,0.465319173179001,0.72727602985543));
#17746=DIRECTION('center_axis',(-1.,0.,0.));
#17747=DIRECTION('ref_axis',(0.,0.707106781186546,-0.707106781186549));
#17748=DIRECTION('',(1.,0.,0.));
#17749=DIRECTION('',(-1.,0.,0.));
#17750=DIRECTION('center_axis',(0.,1.,0.));
#17751=DIRECTION('ref_axis',(-1.,0.,0.));
#17752=DIRECTION('',(0.,0.,1.));
#17753=DIRECTION('',(-1.,0.,0.));
#17754=DIRECTION('',(0.,0.,1.));
#17755=DIRECTION('',(0.881917103688202,0.,0.471404520791021));
#17756=DIRECTION('center_axis',(0.,0.,1.));
#17757=DIRECTION('ref_axis',(-9.51619735392991E-16,1.,0.));
#17758=DIRECTION('',(0.,0.,1.));
#17759=DIRECTION('center_axis',(0.,0.,1.));
#17760=DIRECTION('ref_axis',(-9.51619735392991E-16,1.,0.));
#17761=DIRECTION('',(0.,-0.881917103688202,-0.471404520791021));
#17762=DIRECTION('',(-0.504527148397114,-0.465319173179004,-0.727276029855435));
#17763=DIRECTION('center_axis',(0.,0.,1.));
#17764=DIRECTION('ref_axis',(1.,1.26882631385732E-15,0.));
#17765=DIRECTION('',(0.494871659305391,0.505076272276104,0.70710678118655));
#17766=DIRECTION('center_axis',(0.,0.,-1.));
#17767=DIRECTION('ref_axis',(1.,1.26882631385732E-15,0.));
#17768=DIRECTION('',(-0.505076272276111,-0.494871659305385,-0.70710678118655));
#17769=DIRECTION('center_axis',(0.,0.,1.));
#17770=DIRECTION('ref_axis',(1.,1.26882631385732E-15,0.));
#17771=DIRECTION('',(0.465319173178992,0.504527148397119,0.72727602985544));
#17772=DIRECTION('center_axis',(0.,0.,1.));
#17773=DIRECTION('ref_axis',(1.,0.,0.));
#17774=DIRECTION('',(0.,1.,0.));
#17775=DIRECTION('center_axis',(0.,0.,1.));
#17776=DIRECTION('ref_axis',(1.26882631385732E-15,-1.,0.));
#17777=DIRECTION('',(1.,0.,0.));
#17778=DIRECTION('center_axis',(0.,0.,1.));
#17779=DIRECTION('ref_axis',(-1.,-1.26882631385732E-15,0.));
#17780=DIRECTION('',(0.,-1.,0.));
#17781=DIRECTION('center_axis',(-0.577350269189622,-0.577350269189634,0.577350269189622));
#17782=DIRECTION('ref_axis',(0.707106781186547,0.,0.707106781186547));
#17783=DIRECTION('',(0.,-0.70710678118654,-0.707106781186555));
#17784=DIRECTION('',(-0.707106781186555,0.70710678118654,0.));
#17785=DIRECTION('center_axis',(0.,-0.707106781186555,0.70710678118654));
#17786=DIRECTION('ref_axis',(1.,0.,0.));
#17787=DIRECTION('',(1.,0.,0.));
#17788=DIRECTION('',(0.577350269189628,0.577350269189618,0.577350269189631));
#17789=DIRECTION('center_axis',(0.,-0.707106781186548,0.707106781186548));
#17790=DIRECTION('ref_axis',(1.,0.,0.));
#17791=DIRECTION('',(1.,0.,0.));
#17792=DIRECTION('',(0.,0.707106781186548,0.707106781186548));
#17793=DIRECTION('',(-0.577350269189629,-0.577350269189619,-0.577350269189629));
#17794=DIRECTION('center_axis',(0.,0.,-1.));
#17795=DIRECTION('ref_axis',(1.26882631385732E-15,-1.,0.));
#17796=DIRECTION('',(-0.707106781186548,0.,0.707106781186548));
#17797=DIRECTION('center_axis',(0.,0.,1.));
#17798=DIRECTION('ref_axis',(1.26882631385732E-15,-1.,0.));
#17799=DIRECTION('center_axis',(0.707106781186548,0.,0.707106781186548));
#17800=DIRECTION('ref_axis',(0.707106781186548,0.,-0.707106781186548));
#17801=DIRECTION('',(-0.707106781186548,0.,0.707106781186548));
#17802=DIRECTION('',(0.,1.,0.));
#17803=DIRECTION('center_axis',(0.,0.,-1.));
#17804=DIRECTION('ref_axis',(1.,1.26882631385732E-15,0.));
#17805=DIRECTION('',(0.,-0.707106781186548,0.707106781186548));
#17806=DIRECTION('center_axis',(0.,0.,1.));
#17807=DIRECTION('ref_axis',(1.,1.26882631385732E-15,0.));
#17808=DIRECTION('center_axis',(0.,0.707106781186548,0.707106781186548));
#17809=DIRECTION('ref_axis',(1.,0.,0.));
#17810=DIRECTION('',(0.,-0.707106781186548,0.707106781186548));
#17811=DIRECTION('center_axis',(0.,0.,-1.));
#17812=DIRECTION('ref_axis',(-9.5161973539299E-16,1.,0.));
#17813=DIRECTION('',(0.707106781186549,0.,0.707106781186546));
#17814=DIRECTION('center_axis',(-0.707106781186546,0.,0.707106781186549));
#17815=DIRECTION('ref_axis',(0.707106781186549,0.,0.707106781186546));
#17816=DIRECTION('',(0.707106781186549,0.,0.707106781186546));
#17817=DIRECTION('',(0.,-1.,0.));
#17818=DIRECTION('center_axis',(0.,0.,-1.));
#17819=DIRECTION('ref_axis',(-1.,-1.26882631385732E-15,0.));
#17820=DIRECTION('',(0.,0.707106781186548,0.707106781186548));
#17821=DIRECTION('center_axis',(0.,0.,1.));
#17822=DIRECTION('ref_axis',(-1.,-1.26882631385732E-15,0.));
#17823=DIRECTION('center_axis',(0.,-0.707106781186548,0.707106781186548));
#17824=DIRECTION('ref_axis',(1.,0.,0.));
#17825=DIRECTION('',(1.,0.,0.));
#17826=DIRECTION('',(-0.577350269189632,0.577350269189618,0.577350269189628));
#17827=DIRECTION('center_axis',(0.707106781186541,-0.707106781186554,0.));
#17828=DIRECTION('ref_axis',(0.,0.,-1.));
#17829=DIRECTION('',(0.,0.,-1.));
#17830=DIRECTION('',(0.,0.,1.));
#17831=DIRECTION('center_axis',(-0.70710678118654,-0.707106781186555,0.));
#17832=DIRECTION('ref_axis',(0.,0.,1.));
#17833=DIRECTION('',(0.,0.,1.));
#17834=DIRECTION('',(0.,0.,-1.));
#17835=DIRECTION('center_axis',(0.,0.,1.));
#17836=DIRECTION('ref_axis',(1.,1.26882631385732E-15,0.));
#17837=DIRECTION('',(0.,0.,1.));
#17838=DIRECTION('center_axis',(1.,0.,0.));
#17839=DIRECTION('ref_axis',(0.,1.,0.));
#17840=DIRECTION('',(0.,0.,1.));
#17841=DIRECTION('',(0.,-0.881917103688205,0.471404520791017));
#17842=DIRECTION('',(0.,-1.,0.));
#17843=DIRECTION('center_axis',(0.,0.,1.));
#17844=DIRECTION('ref_axis',(1.26882631385732E-15,-1.,0.));
#17845=DIRECTION('',(0.,0.,1.));
#17846=DIRECTION('center_axis',(0.,0.,-1.));
#17847=DIRECTION('ref_axis',(1.26882631385732E-15,-1.,0.));
#17848=DIRECTION('center_axis',(-1.,0.,0.));
#17849=DIRECTION('ref_axis',(0.,0.,-1.));
#17850=DIRECTION('center_axis',(1.,0.,0.));
#17851=DIRECTION('ref_axis',(0.,0.,1.));
#17852=DIRECTION('',(0.,0.881917103688198,-0.471404520791029));
#17853=DIRECTION('',(-0.881917103688201,0.,0.471404520791024));
#17854=DIRECTION('',(0.504527148397123,0.46531917317901,-0.727276029855426));
#17855=DIRECTION('center_axis',(0.,0.,1.));
#17856=DIRECTION('ref_axis',(-1.,-1.26882631385732E-15,0.));
#17857=DIRECTION('',(-0.49487165930539,-0.505076272276101,0.707106781186553));
#17858=DIRECTION('center_axis',(0.,0.,-1.));
#17859=DIRECTION('ref_axis',(-1.,-1.26882631385732E-15,0.));
#17860=DIRECTION('',(0.505076272276103,0.494871659305383,-0.707106781186557));
#17861=DIRECTION('',(-0.465319173178996,-0.504527148397133,0.727276029855427));
#17862=DIRECTION('center_axis',(0.,-1.,0.));
#17863=DIRECTION('ref_axis',(-0.707106781186546,0.,-0.707106781186549));
#17864=DIRECTION('',(0.,1.,0.));
#17865=DIRECTION('center_axis',(-1.,0.,0.));
#17866=DIRECTION('ref_axis',(0.,-1.,0.));
#17867=DIRECTION('',(0.,0.,1.));
#17868=DIRECTION('center_axis',(0.,0.,1.));
#17869=DIRECTION('ref_axis',(-1.,-1.26882631385732E-15,0.));
#17870=DIRECTION('',(0.,0.,1.));
#17871=DIRECTION('',(-0.881917103688201,0.,-0.471404520791023));
#17872=DIRECTION('',(-0.465319173178989,0.504527148397135,-0.727276029855431));
#17873=DIRECTION('center_axis',(0.,0.,1.));
#17874=DIRECTION('ref_axis',(1.26882631385732E-15,-1.,0.));
#17875=DIRECTION('',(0.5050762722761,-0.494871659305393,0.707106781186552));
#17876=DIRECTION('',(-0.494871659305393,0.5050762722761,-0.707106781186552));
#17877=DIRECTION('',(0.50452714839712,-0.465319173179011,0.727276029855427));
#17878=DIRECTION('center_axis',(0.,1.,0.));
#17879=DIRECTION('ref_axis',(0.707106781186548,0.,-0.707106781186548));
#17880=DIRECTION('center_axis',(1.,0.,0.));
#17881=DIRECTION('ref_axis',(0.,-0.707106781186548,-0.707106781186548));
#17882=DIRECTION('',(-1.,0.,0.));
#17883=DIRECTION('center_axis',(0.,-1.,0.));
#17884=DIRECTION('ref_axis',(1.,0.,0.));
#17885=DIRECTION('center_axis',(0.,0.,-1.));
#17886=DIRECTION('ref_axis',(9.86864910777915E-16,-1.,0.));
#17887=DIRECTION('',(0.,0.,-1.));
#17888=DIRECTION('center_axis',(0.,0.,-1.));
#17889=DIRECTION('ref_axis',(9.86864910777915E-16,-1.,0.));
#17890=DIRECTION('center_axis',(1.,0.,0.));
#17891=DIRECTION('ref_axis',(0.,-1.,0.));
#17892=DIRECTION('',(0.,0.,-1.));
#17893=DIRECTION('',(0.,-1.,0.));
#17894=DIRECTION('center_axis',(0.,0.,-1.));
#17895=DIRECTION('ref_axis',(1.,3.94745964311165E-15,0.));
#17896=DIRECTION('',(0.,0.,-1.));
#17897=DIRECTION('center_axis',(0.,0.,-1.));
#17898=DIRECTION('ref_axis',(1.,3.94745964311165E-15,0.));
#17899=DIRECTION('center_axis',(0.,1.,0.));
#17900=DIRECTION('ref_axis',(1.,0.,0.));
#17901=DIRECTION('',(1.,0.,0.));
#17902=DIRECTION('center_axis',(0.,0.,1.));
#17903=DIRECTION('ref_axis',(1.,0.,0.));
#29366=CARTESIAN_POINT('',(0.,0.,0.));
#29367=CARTESIAN_POINT('Origin',(25.7,-73.75,-60.25));
#29368=CARTESIAN_POINT('',(-5.8,-73.5,-60.5));
#29369=CARTESIAN_POINT('',(-5.8,-74.,-60.));
#29370=CARTESIAN_POINT('',(-5.8,-73.5,-60.5));
#29371=CARTESIAN_POINT('',(6.7,-74.,-60.));
#29372=CARTESIAN_POINT('',(25.7,-74.,-60.));
#29373=CARTESIAN_POINT('',(23.7,-74.,-60.));
#29374=CARTESIAN_POINT('',(15.2,-74.,-60.));
#29375=CARTESIAN_POINT('',(36.2,-74.,-60.));
#29376=CARTESIAN_POINT('',(25.7,-74.,-60.));
#29377=CARTESIAN_POINT('',(36.2,-73.5,-60.5));
#29378=CARTESIAN_POINT('',(36.2,-74.,-60.));
#29379=CARTESIAN_POINT('',(25.7,-73.5,-60.5));
#29380=CARTESIAN_POINT('Origin',(-5.8,-69.,-60.25));
#29381=CARTESIAN_POINT('',(-10.3,-69.,-60.5));
#29382=CARTESIAN_POINT('',(-10.8,-69.,-60.));
#29383=CARTESIAN_POINT('',(-10.3,-69.,-60.5));
#29384=CARTESIAN_POINT('Origin',(-5.8,-69.,-60.));
#29385=CARTESIAN_POINT('Origin',(-5.8,-69.,-60.5));
#29386=CARTESIAN_POINT('Origin',(-10.55,-61.,-60.25));
#29387=CARTESIAN_POINT('',(-10.3,-37.,-60.5));
#29388=CARTESIAN_POINT('',(-10.8,-37.,-60.));
#29389=CARTESIAN_POINT('',(-10.3,-37.,-60.5));
#29390=CARTESIAN_POINT('',(-10.8,-61.,-60.));
#29391=CARTESIAN_POINT('',(-10.3,-61.,-60.5));
#29392=CARTESIAN_POINT('Origin',(-5.79999999999999,-37.,-60.25));
#29393=CARTESIAN_POINT('',(-5.8,-32.5,-60.5));
#29394=CARTESIAN_POINT('',(-5.8,-32.,-60.));
#29395=CARTESIAN_POINT('',(-5.8,-32.5,-60.5));
#29396=CARTESIAN_POINT('Origin',(-5.79999999999999,-37.,-60.));
#29397=CARTESIAN_POINT('Origin',(-5.79999999999999,-37.,-60.5));
#29398=CARTESIAN_POINT('Origin',(4.7,-32.25,-60.25));
#29399=CARTESIAN_POINT('',(36.2,-32.5,-60.5));
#29400=CARTESIAN_POINT('',(36.2,-32.,-60.));
#29401=CARTESIAN_POINT('',(36.2,-32.5,-60.5));
#29402=CARTESIAN_POINT('',(4.7,-32.,-60.));
#29403=CARTESIAN_POINT('',(4.7,-32.5,-60.5));
#29404=CARTESIAN_POINT('Origin',(36.2,-37.,-60.25));
#29405=CARTESIAN_POINT('',(40.7,-37.,-60.5));
#29406=CARTESIAN_POINT('',(41.2,-37.,-60.));
#29407=CARTESIAN_POINT('',(40.7,-37.,-60.5));
#29408=CARTESIAN_POINT('Origin',(36.2,-37.,-60.));
#29409=CARTESIAN_POINT('Origin',(36.2,-37.,-60.5));
#29410=CARTESIAN_POINT('Origin',(40.95,-45.,-60.25));
#29411=CARTESIAN_POINT('',(40.7,-69.,-60.5));
#29412=CARTESIAN_POINT('',(41.2,-69.,-60.));
#29413=CARTESIAN_POINT('',(40.7,-69.,-60.5));
#29414=CARTESIAN_POINT('',(41.2,-45.,-60.));
#29415=CARTESIAN_POINT('',(40.7,-45.,-60.5));
#29416=CARTESIAN_POINT('Origin',(36.2,-69.,-60.25));
#29417=CARTESIAN_POINT('Origin',(36.2,-69.,-60.));
#29418=CARTESIAN_POINT('Origin',(36.2,-69.,-60.5));
#29419=CARTESIAN_POINT('Origin',(15.2,-53.,-60.));
#29420=CARTESIAN_POINT('',(24.2,-74.5,-60.));
#29421=CARTESIAN_POINT('',(16.45,-66.7499999999999,-60.));
#29422=CARTESIAN_POINT('',(24.2,-75.5,-60.));
#29423=CARTESIAN_POINT('',(24.2,-63.5,-60.));
#29424=CARTESIAN_POINT('',(36.2,-75.5,-60.));
#29425=CARTESIAN_POINT('',(4.7,-75.5,-60.));
#29426=CARTESIAN_POINT('',(42.7,-69.,-60.));
#29427=CARTESIAN_POINT('Origin',(36.2,-69.,-60.));
#29428=CARTESIAN_POINT('',(42.7,-37.,-60.));
#29429=CARTESIAN_POINT('',(42.7,-61.,-60.));
#29430=CARTESIAN_POINT('',(36.2,-30.5,-60.));
#29431=CARTESIAN_POINT('Origin',(36.2,-37.,-60.));
#29432=CARTESIAN_POINT('',(-5.8,-30.5,-60.));
#29433=CARTESIAN_POINT('',(25.7,-30.5,-60.));
#29434=CARTESIAN_POINT('',(-12.3,-37.,-60.));
#29435=CARTESIAN_POINT('Origin',(-5.79999999999999,-37.,-60.));
#29436=CARTESIAN_POINT('',(-12.3,-69.,-60.));
#29437=CARTESIAN_POINT('',(-12.3,-45.,-60.));
#29438=CARTESIAN_POINT('',(-5.8,-75.5,-60.));
#29439=CARTESIAN_POINT('Origin',(-5.8,-69.,-60.));
#29440=CARTESIAN_POINT('',(6.2,-75.5,-60.));
#29441=CARTESIAN_POINT('',(4.7,-75.5,-60.));
#29442=CARTESIAN_POINT('',(6.2,-74.5,-60.));
#29443=CARTESIAN_POINT('',(6.2,-63.5,-60.));
#29444=CARTESIAN_POINT('',(13.95,-66.7499999999999,-60.));
#29445=CARTESIAN_POINT('Origin',(-5.79999999999999,-37.,-60.));
#29446=CARTESIAN_POINT('',(-10.3,-37.,-79.5));
#29447=CARTESIAN_POINT('',(-10.3,-37.,-60.));
#29448=CARTESIAN_POINT('',(-5.8,-32.5,-79.5));
#29449=CARTESIAN_POINT('Origin',(-5.79999999999999,-37.,-79.5));
#29450=CARTESIAN_POINT('',(-5.8,-32.5,-60.));
#29451=CARTESIAN_POINT('Origin',(-10.3,-69.,-60.));
#29452=CARTESIAN_POINT('',(-10.3,-69.,-79.5));
#29453=CARTESIAN_POINT('',(-10.3,-69.,-60.));
#29454=CARTESIAN_POINT('',(-10.3,-37.,-79.5));
#29455=CARTESIAN_POINT('Origin',(-5.8,-69.,-60.));
#29456=CARTESIAN_POINT('',(-5.8,-73.5,-79.5));
#29457=CARTESIAN_POINT('',(-5.8,-73.5,-60.));
#29458=CARTESIAN_POINT('Origin',(-5.8,-69.,-79.5));
#29459=CARTESIAN_POINT('Origin',(36.2,-73.5,-60.));
#29460=CARTESIAN_POINT('',(36.2,-73.5,-79.5));
#29461=CARTESIAN_POINT('',(36.2,-73.5,-60.));
#29462=CARTESIAN_POINT('',(-5.8,-73.5,-79.5));
#29463=CARTESIAN_POINT('Origin',(23.7,-74.5,-12.));
#29464=CARTESIAN_POINT('',(23.7,-74.,-12.5));
#29465=CARTESIAN_POINT('',(24.2,-74.5,-12.5));
#29466=CARTESIAN_POINT('',(23.7,-74.,-12.5));
#29467=CARTESIAN_POINT('',(23.7,-74.5,-12.));
#29468=CARTESIAN_POINT('',(23.7,-74.5,-12.));
#29469=CARTESIAN_POINT('',(24.2,-74.5,-12.5));
#29470=CARTESIAN_POINT('Origin',(19.7,-74.25,-12.25));
#29471=CARTESIAN_POINT('',(6.45,-74.25,-12.25));
#29472=CARTESIAN_POINT('',(6.7,-74.5,-12.));
#29473=CARTESIAN_POINT('',(8.61666666666665,-76.4166666666667,-10.0833333333334));
#29474=CARTESIAN_POINT('',(19.7,-74.5,-12.));
#29475=CARTESIAN_POINT('',(6.7,-74.,-12.5));
#29476=CARTESIAN_POINT('',(19.7,-74.,-12.5));
#29477=CARTESIAN_POINT('',(10.8666666666666,-69.8333333333333,-16.6666666666666));
#29478=CARTESIAN_POINT('Origin',(23.95,-74.,-12.25));
#29479=CARTESIAN_POINT('',(23.95,-75.75,-12.25));
#29480=CARTESIAN_POINT('',(24.2,-75.5,-12.5));
#29481=CARTESIAN_POINT('',(34.5333333333335,-65.1666666666667,-22.8333333333335));
#29482=CARTESIAN_POINT('',(24.2,-74.,-12.5));
#29483=CARTESIAN_POINT('',(23.7,-75.5,-12.));
#29484=CARTESIAN_POINT('',(23.7,-74.,-12.));
#29485=CARTESIAN_POINT('',(21.2,-73.,-9.49999999999997));
#29486=CARTESIAN_POINT('Origin',(23.95,-74.25,-52.5));
#29487=CARTESIAN_POINT('',(23.7,-74.,-52.5));
#29488=CARTESIAN_POINT('',(24.2,-74.5,-52.5));
#29489=CARTESIAN_POINT('Origin',(24.2,-74.,-12.));
#29490=CARTESIAN_POINT('',(6.7,-75.5,-12.));
#29491=CARTESIAN_POINT('',(6.7,-74.,-12.));
#29492=CARTESIAN_POINT('',(9.2,-75.5,-12.));
#29493=CARTESIAN_POINT('Origin',(6.45,-74.,-12.25));
#29494=CARTESIAN_POINT('',(6.2,-74.5,-12.5));
#29495=CARTESIAN_POINT('',(4.28333333333335,-76.4166666666667,-14.4166666666666));
#29496=CARTESIAN_POINT('',(6.2,-75.5,-12.5));
#29497=CARTESIAN_POINT('',(6.2,-74.,-12.5));
#29498=CARTESIAN_POINT('',(6.2,-75.5,-12.5));
#29499=CARTESIAN_POINT('Origin',(6.45,-74.25,-25.5));
#29500=CARTESIAN_POINT('',(6.7,-74.,-25.5));
#29501=CARTESIAN_POINT('',(6.2,-74.5,-25.5));
#29502=CARTESIAN_POINT('Origin',(15.2,-74.,-39.));
#29503=CARTESIAN_POINT('Ctrl Pts',(-5.56630111765684,-30.048846456053,-80.4393174796692));
#29504=CARTESIAN_POINT('Ctrl Pts',(-5.55472999163838,-30.0474878607419,
-80.4332835106634));
#29505=CARTESIAN_POINT('Ctrl Pts',(-5.50914704734725,-30.0412161151931,
-80.4097058743082));
#29506=CARTESIAN_POINT('Ctrl Pts',(-5.26592539574766,-30.018413630151,-80.2818322468851));
#29507=CARTESIAN_POINT('Ctrl Pts',(-5.03984528472998,-30.0051078595377,
-80.1608659535269));
#29508=CARTESIAN_POINT('Ctrl Pts',(-4.79674507928722,-29.9990490307073,
-80.0305394911781));
#29509=CARTESIAN_POINT('Ctrl Pts',(-4.75094774329034,-30.,-80.006159003494));
#29510=CARTESIAN_POINT('Ctrl Pts',(-4.73933982822015,-30.,-80.));
#29511=CARTESIAN_POINT('Ctrl Pts',(-5.72305909304156,-30.033897250275,-80.1460536871276));
#29512=CARTESIAN_POINT('Ctrl Pts',(-5.71422864812372,-30.0331851743567,
-80.1414222172682));
#29513=CARTESIAN_POINT('Ctrl Pts',(-5.68538075880276,-30.029214011803,-80.126606885425));
#29514=CARTESIAN_POINT('Ctrl Pts',(-5.48880222005144,-30.0103524135108,
-80.0234452250129));
#29515=CARTESIAN_POINT('Ctrl Pts',(-5.32713234249905,-30.0016369910093,
-79.9366792528958));
#29516=CARTESIAN_POINT('Ctrl Pts',(-5.13072308176098,-29.998410805748,-79.8311710354903));
#29517=CARTESIAN_POINT('Ctrl Pts',(-5.10173254804783,-30.,-79.8157122686222));
#29518=CARTESIAN_POINT('Ctrl Pts',(-5.09289321881343,-30.,-79.8110177634954));
#29519=CARTESIAN_POINT('Ctrl Pts',(-5.87981706842629,-30.018948044497,-79.8527898945859));
#29520=CARTESIAN_POINT('Ctrl Pts',(-5.87375891162897,-30.0186527919516,
-79.8495895275592));
#29521=CARTESIAN_POINT('Ctrl Pts',(-5.8439723661837,-30.0162635432914,-79.8337973075619));
#29522=CARTESIAN_POINT('Ctrl Pts',(-5.727605526545,-30.0100867792541,-79.7718561188082));
#29523=CARTESIAN_POINT('Ctrl Pts',(-5.59851606708718,-30.0033535127243,
-79.7031093748739));
#29524=CARTESIAN_POINT('Ctrl Pts',(-5.48232352746253,-30.000714223928,-79.6411500710076));
#29525=CARTESIAN_POINT('Ctrl Pts',(-5.45251735280532,-30.,-79.6252655337503));
#29526=CARTESIAN_POINT('Ctrl Pts',(-5.44644660940672,-30.,-79.6220355269908));
#29527=CARTESIAN_POINT('Ctrl Pts',(-6.03657504381102,-30.0039988387189,
-79.5595261020443));
#29528=CARTESIAN_POINT('Ctrl Pts',(-6.03327514811522,-30.0038872502628,
-79.5577612253643));
#29529=CARTESIAN_POINT('Ctrl Pts',(-6.02026555880084,-30.0033696172087,
-79.5508019948342));
#29530=CARTESIAN_POINT('Ctrl Pts',(-5.95065272607528,-30.0014965556721,
-79.5135781548536));
#29531=CARTESIAN_POINT('Ctrl Pts',(-5.88593766744229,-30.0004169765915,
-79.4789879704714));
#29532=CARTESIAN_POINT('Ctrl Pts',(-5.81635283613372,-29.9999223146288,
-79.4417957477402));
#29533=CARTESIAN_POINT('Ctrl Pts',(-5.8033021575628,-30.,-79.4348187988785));
#29534=CARTESIAN_POINT('Ctrl Pts',(-5.8,-30.,-79.4330532904862));
#29535=CARTESIAN_POINT('',(-4.73933982822015,-30.,-80.));
#29536=CARTESIAN_POINT('',(-5.56630111765684,-30.048846456053,-80.4393174796692));
#29537=CARTESIAN_POINT('Ctrl Pts',(-4.73933982822015,-30.,-80.));
#29538=CARTESIAN_POINT('Ctrl Pts',(-4.74144196548162,-30.,-80.0011153657362));
#29539=CARTESIAN_POINT('Ctrl Pts',(-4.74354800689035,-30.0000008803716,
-80.0022328244698));
#29540=CARTESIAN_POINT('Ctrl Pts',(-4.74582631569054,-30.000002963202,-80.0034427894735));
#29541=CARTESIAN_POINT('Ctrl Pts',(-4.74816258095287,-30.0000050990163,
-80.0046835340147));
#29542=CARTESIAN_POINT('Ctrl Pts',(-4.75067986365268,-30.0000084969638,
-80.0060214841799));
#29543=CARTESIAN_POINT('Ctrl Pts',(-4.75351150864003,-30.0000141688287,
-80.007528287592));
#29544=CARTESIAN_POINT('Ctrl Pts',(-4.756425520977,-30.0000200056777,-80.0090789211466));
#29545=CARTESIAN_POINT('Ctrl Pts',(-4.75967230457741,-30.0000282443224,
-80.0108082969316));
#29546=CARTESIAN_POINT('Ctrl Pts',(-4.7633488278572,-30.0000407594512,-80.0127685607417));
#29547=CARTESIAN_POINT('Ctrl Pts',(-4.76722661255211,-30.0000539596872,
-80.0148361339413));
#29548=CARTESIAN_POINT('Ctrl Pts',(-4.77158245475638,-30.0000719133563,
-80.0171605566096));
#29549=CARTESIAN_POINT('Ctrl Pts',(-4.77647810826652,-30.0000977659287,
-80.0197750892952));
#29550=CARTESIAN_POINT('Ctrl Pts',(-4.78159298377548,-30.000124776151,-80.022506697889));
#29551=CARTESIAN_POINT('Ctrl Pts',(-4.78729688562401,-30.0001604227472,
-80.0255548684521));
#29552=CARTESIAN_POINT('Ctrl Pts',(-4.79360683616279,-30.0002092303521,
-80.0289288373614));
#29553=CARTESIAN_POINT('Ctrl Pts',(-4.80027903556804,-30.0002608399599,
-80.0324965029417));
#29554=CARTESIAN_POINT('Ctrl Pts',(-4.80762859173676,-30.0003272062035,
-80.0364283036621));
#29555=CARTESIAN_POINT('Ctrl Pts',(-4.81562085393833,-30.0004142810683,
-80.0407056831963));
#29556=CARTESIAN_POINT('Ctrl Pts',(-4.8242508272187,-30.000508303729,-80.0453243593808));
#29557=CARTESIAN_POINT('Ctrl Pts',(-4.83362976955803,-30.0006265572524,
-80.0503457549901));
#29558=CARTESIAN_POINT('Ctrl Pts',(-4.84365690035937,-30.0007762101847,
-80.0557156911153));
#29559=CARTESIAN_POINT('Ctrl Pts',(-4.85499010112282,-30.0009453559513,
-80.0617850807941));
#29560=CARTESIAN_POINT('Ctrl Pts',(-4.86715064877518,-30.0011547962203,
-80.0682993507869));
#29561=CARTESIAN_POINT('Ctrl Pts',(-4.87993057163511,-30.0014122484325,
-80.0751465187787));
#29562=CARTESIAN_POINT('Ctrl Pts',(-4.89907991110256,-30.0017980128745,
-80.0854062633565));
#29563=CARTESIAN_POINT('Ctrl Pts',(-4.91961655620725,-30.0022930469157,
-80.0964116614511));
#29564=CARTESIAN_POINT('Ctrl Pts',(-4.94072156757471,-30.0029030737397,
-80.1077212473092));
#29565=CARTESIAN_POINT('Ctrl Pts',(-4.95561362249427,-30.0033335190405,
-80.1157014834145));
#29566=CARTESIAN_POINT('Ctrl Pts',(-4.97078474057349,-30.003820567599,-80.1238310489004));
#29567=CARTESIAN_POINT('Ctrl Pts',(-4.98596678089125,-30.0043584577033,
-80.1319652782344));
#29568=CARTESIAN_POINT('Ctrl Pts',(-4.99882878382487,-30.0048141503476,
-80.1388564785847));
#29569=CARTESIAN_POINT('Ctrl Pts',(-5.01169802485068,-30.0053061295215,
-80.1457507055734));
#29570=CARTESIAN_POINT('Ctrl Pts',(-5.02444777245903,-30.0058286173219,
-80.1525794760373));
#29571=CARTESIAN_POINT('Ctrl Pts',(-5.03614342853803,-30.0063079081916,
-80.1588436746115));
#29572=CARTESIAN_POINT('Ctrl Pts',(-5.04773815869922,-30.0068127545887,
-80.1650525968365));
#29573=CARTESIAN_POINT('Ctrl Pts',(-5.05917370952967,-30.0073386464146,
-80.1711745598128));
#29574=CARTESIAN_POINT('Ctrl Pts',(-5.06994987742711,-30.0078342149006,
-80.1769435255471));
#29575=CARTESIAN_POINT('Ctrl Pts',(-5.08058442371394,-30.0083483842256,
-80.1826351325825));
#29576=CARTESIAN_POINT('Ctrl Pts',(-5.09106981935722,-30.0088787394278,
-80.1882448556992));
#29577=CARTESIAN_POINT('Ctrl Pts',(-5.10108922385955,-30.0093855246251,
-80.1936052719358));
#29578=CARTESIAN_POINT('Ctrl Pts',(-5.11097222934838,-30.0099070182464,
-80.1988908141908));
#29579=CARTESIAN_POINT('Ctrl Pts',(-5.12075449580623,-30.0104435082543,
-80.2041199797976));
#29580=CARTESIAN_POINT('Ctrl Pts',(-5.13066213607484,-30.0109868741531,
-80.2094161646808));
#29581=CARTESIAN_POINT('Ctrl Pts',(-5.14046580534474,-30.0115455183055,
-80.2146541901608));
#29582=CARTESIAN_POINT('Ctrl Pts',(-5.15025372270428,-30.0121235896603,
-80.2198803702353));
#29583=CARTESIAN_POINT('Ctrl Pts',(-5.15964979940463,-30.0126785190276,
-80.2248973301284));
#29584=CARTESIAN_POINT('Ctrl Pts',(-5.16903937197897,-30.0132518166605,
-80.2299076190967));
#29585=CARTESIAN_POINT('Ctrl Pts',(-5.17851048157321,-30.0138491970066,
-80.2349574169266));
#29586=CARTESIAN_POINT('Ctrl Pts',(-5.18857236361835,-30.0144838397081,
-80.2403222022889));
#29587=CARTESIAN_POINT('Ctrl Pts',(-5.1987263082372,-30.0151457246997,-80.2457315928303));
#29588=CARTESIAN_POINT('Ctrl Pts',(-5.20902221469754,-30.0158395174066,
-80.2512114235356));
#29589=CARTESIAN_POINT('Ctrl Pts',(-5.21965634603708,-30.0165561014972,
-80.2568712689959));
#29590=CARTESIAN_POINT('Ctrl Pts',(-5.23044154664282,-30.0173067739427,
-80.2626060532407));
#29591=CARTESIAN_POINT('Ctrl Pts',(-5.24137829908528,-30.0180935545994,
-80.268415427425));
#29592=CARTESIAN_POINT('Ctrl Pts',(-5.25298609557392,-30.0189286095934,
-80.2745812461735));
#29593=CARTESIAN_POINT('Ctrl Pts',(-5.26476428837502,-30.0198044087532,
-80.2808309052075));
#29594=CARTESIAN_POINT('Ctrl Pts',(-5.2766581599697,-30.0207189336069,-80.2871349164031));
#29595=CARTESIAN_POINT('Ctrl Pts',(-5.28959276745022,-30.0217134810862,
-80.2939905403031));
#29596=CARTESIAN_POINT('Ctrl Pts',(-5.30266369650548,-30.0227539199694,
-80.3009101655443));
#29597=CARTESIAN_POINT('Ctrl Pts',(-5.31574313110297,-30.0238311868593,
-80.3078259605203));
#29598=CARTESIAN_POINT('Ctrl Pts',(-5.33103182386516,-30.0250904157947,
-80.3159099081716));
#29599=CARTESIAN_POINT('Ctrl Pts',(-5.34633124270374,-30.0264001451606,
-80.3239880989655));
#29600=CARTESIAN_POINT('Ctrl Pts',(-5.36137151862682,-30.0277348059174,
-80.331918671078));
#29601=CARTESIAN_POINT('Ctrl Pts',(-5.3804794850386,-30.0294304299233,-80.3419940916572));
#29602=CARTESIAN_POINT('Ctrl Pts',(-5.39916371312678,-30.0311663675709,
-80.3518282328887));
#29603=CARTESIAN_POINT('Ctrl Pts',(-5.41681836687482,-30.032869487213,-80.3611060033595));
#29604=CARTESIAN_POINT('Ctrl Pts',(-5.42939363939264,-30.0340826060843,
-80.3677144870881));
#29605=CARTESIAN_POINT('Ctrl Pts',(-5.44144478107398,-30.0352784415749,
-80.3740398610588));
#29606=CARTESIAN_POINT('Ctrl Pts',(-5.45277520515776,-30.0364281559369,
-80.3799810695321));
#29607=CARTESIAN_POINT('Ctrl Pts',(-5.46295272876472,-30.0374608838361,
-80.3853177444037));
#29608=CARTESIAN_POINT('Ctrl Pts',(-5.47254808492725,-30.0384562049433,
-80.3903441398836));
#29609=CARTESIAN_POINT('Ctrl Pts',(-5.48145278810254,-30.0393952767108,
-80.3950052139099));
#29610=CARTESIAN_POINT('Ctrl Pts',(-5.48976990866469,-30.0402723832188,
-80.3993587239443));
#29611=CARTESIAN_POINT('Ctrl Pts',(-5.49748410046507,-30.0411003010874,
-80.4033933349473));
#29612=CARTESIAN_POINT('Ctrl Pts',(-5.50454551684857,-30.0418676601101,
-80.4070844377734));
#29613=CARTESIAN_POINT('Ctrl Pts',(-5.51126001057488,-30.042597319298,-80.4105941991899));
#29614=CARTESIAN_POINT('Ctrl Pts',(-5.51738399137094,-30.0432721483508,
-80.413793229439));
#29615=CARTESIAN_POINT('Ctrl Pts',(-5.52291574173486,-30.0438874474019,
-80.4166817509419));
#29616=CARTESIAN_POINT('Ctrl Pts',(-5.5284930595309,-30.0445078149387,-80.419594066452));
#29617=CARTESIAN_POINT('Ctrl Pts',(-5.53346765422382,-30.0450675579802,
-80.422190383135));
#29618=CARTESIAN_POINT('Ctrl Pts',(-5.53788859927536,-30.0455685938731,
-80.4244972069931));
#29619=CARTESIAN_POINT('Ctrl Pts',(-5.5419030547062,-30.0460235613604,-80.4265919268906));
#29620=CARTESIAN_POINT('Ctrl Pts',(-5.54546126449629,-30.0464301580792,
-80.4284480840646));
#29621=CARTESIAN_POINT('Ctrl Pts',(-5.54864302299335,-30.0467956231858,
-80.4301077334735));
#29622=CARTESIAN_POINT('Ctrl Pts',(-5.55175296235284,-30.0471528389582,
-80.4317299210232));
#29623=CARTESIAN_POINT('Ctrl Pts',(-5.55450305873677,-30.0474707401459,
-80.4331642707516));
#29624=CARTESIAN_POINT('Ctrl Pts',(-5.55701120543205,-30.047761872528,-80.4344724313979));
#29625=CARTESIAN_POINT('Ctrl Pts',(-5.5594471567617,-30.0480446248546,-80.4357429374937));
#29626=CARTESIAN_POINT('Ctrl Pts',(-5.56165478585712,-30.0483021202198,
-80.4368943615289));
#29627=CARTESIAN_POINT('Ctrl Pts',(-5.56378554069762,-30.0485515407009,
-80.4380056057852));
#29628=CARTESIAN_POINT('Ctrl Pts',(-5.56463185204192,-30.0486506076507,
-80.4384469792378));
#29629=CARTESIAN_POINT('Ctrl Pts',(-5.56546653509834,-30.0487484655939,
-80.4388822717834));
#29630=CARTESIAN_POINT('Ctrl Pts',(-5.56630111765683,-30.048846456053,-80.4393174796692));
#29631=CARTESIAN_POINT('',(-6.03657504381102,-30.0039988387189,-79.5595261020443));
#29632=CARTESIAN_POINT('Ctrl Pts',(-6.03657504381102,-30.0039988387189,
-79.5595261020443));
#29633=CARTESIAN_POINT('Ctrl Pts',(-5.87981706842629,-30.018948044497,-79.8527898945859));
#29634=CARTESIAN_POINT('Ctrl Pts',(-5.72305909304156,-30.033897250275,-80.1460536871276));
#29635=CARTESIAN_POINT('Ctrl Pts',(-5.56630111765684,-30.048846456053,-80.4393174796692));
#29636=CARTESIAN_POINT('',(-5.8,-30.,-79.4330532904862));
#29637=CARTESIAN_POINT('Ctrl Pts',(-6.03657504381102,-30.0039988387189,
-79.5595261020443));
#29638=CARTESIAN_POINT('Ctrl Pts',(-6.03574564719913,-30.0039707920484,
-79.5590825174968));
#29639=CARTESIAN_POINT('Ctrl Pts',(-6.03491215932269,-30.0039427389739,
-79.5586367469676));
#29640=CARTESIAN_POINT('Ctrl Pts',(-6.03395240733885,-30.0039106444314,
-79.5581234464649));
#29641=CARTESIAN_POINT('Ctrl Pts',(-6.03295612114493,-30.0038773281683,
-79.5575906065097));
#29642=CARTESIAN_POINT('Ctrl Pts',(-6.03182396197816,-30.0038396613357,
-79.5569850974549));
#29643=CARTESIAN_POINT('Ctrl Pts',(-6.03047057385369,-30.0037950777162,
-79.5562612724383));
#29644=CARTESIAN_POINT('Ctrl Pts',(-6.02905379370678,-30.0037484058224,
-79.5555035438202));
#29645=CARTESIAN_POINT('Ctrl Pts',(-6.02739480822809,-30.0036941607515,
-79.5546162808493));
#29646=CARTESIAN_POINT('Ctrl Pts',(-6.02544771415954,-30.0036314185014,
-79.5535749449113));
#29647=CARTESIAN_POINT('Ctrl Pts',(-6.02338219594345,-30.003564860207,-79.5524702739127));
#29648=CARTESIAN_POINT('Ctrl Pts',(-6.02099276816558,-30.0034887568951,
-79.5511923847346));
#29649=CARTESIAN_POINT('Ctrl Pts',(-6.01827775435437,-30.0034040546882,
-79.5497404011225));
#29650=CARTESIAN_POINT('Ctrl Pts',(-6.01532769210741,-30.0033120195088,
-79.5481627141069));
#29651=CARTESIAN_POINT('Ctrl Pts',(-6.01199369456653,-30.0032098704196,
-79.5463797332273));
#29652=CARTESIAN_POINT('Ctrl Pts',(-6.00832872223355,-30.0031007479389,
-79.5444198111003));
#29653=CARTESIAN_POINT('Ctrl Pts',(-6.00402471448509,-30.0029725985398,
-79.5421181511546));
#29654=CARTESIAN_POINT('Ctrl Pts',(-5.99926505507077,-30.0028349230635,
-79.5395728983283));
#29655=CARTESIAN_POINT('Ctrl Pts',(-5.99419984919499,-30.0026943457805,
-79.5368643656081));
#29656=CARTESIAN_POINT('Ctrl Pts',(-5.98739362888286,-30.0025054492218,
-79.5332248550199));
#29657=CARTESIAN_POINT('Ctrl Pts',(-5.98004189473503,-30.0023117546125,
-79.529293835965));
#29658=CARTESIAN_POINT('Ctrl Pts',(-5.9725699777804,-30.0021274945332,-79.5252987934978));
#29659=CARTESIAN_POINT('Ctrl Pts',(-5.96758546735511,-30.0020045747668,
-79.5226337035419));
#29660=CARTESIAN_POINT('Ctrl Pts',(-5.96254896392867,-30.0018857753864,
-79.5199409169067));
#29661=CARTESIAN_POINT('Ctrl Pts',(-5.95756360394063,-30.0017735310499,
-79.5172755775885));
#29662=CARTESIAN_POINT('Ctrl Pts',(-5.95308502270938,-30.0016726967311,
-79.5148811790548));
#29663=CARTESIAN_POINT('Ctrl Pts',(-5.94864830234915,-30.0015771320006,
-79.5125092444795));
#29664=CARTESIAN_POINT('Ctrl Pts',(-5.94429524911591,-30.0014873808014,
-79.5101821179178));
#29665=CARTESIAN_POINT('Ctrl Pts',(-5.94022891457763,-30.0014035411647,
-79.5080082701366));
#29666=CARTESIAN_POINT('Ctrl Pts',(-5.93623596369729,-30.0013247573059,
-79.5058737224368));
#29667=CARTESIAN_POINT('Ctrl Pts',(-5.93231359137331,-30.0012506036051,
-79.5037769652748));
#29668=CARTESIAN_POINT('Ctrl Pts',(-5.92852559777125,-30.0011789903769,
-79.5017520420756));
#29669=CARTESIAN_POINT('Ctrl Pts',(-5.92480383064746,-30.0011116815999,
-79.4997625786459));
#29670=CARTESIAN_POINT('Ctrl Pts',(-5.92110444095789,-30.0010476702309,
-79.4977851219757));
#29671=CARTESIAN_POINT('Ctrl Pts',(-5.91728378123075,-30.0009815604993,
-79.4957428421144));
#29672=CARTESIAN_POINT('Ctrl Pts',(-5.91348056649595,-30.0009188424662,
-79.4937099346464));
#29673=CARTESIAN_POINT('Ctrl Pts',(-5.90962244959741,-30.0008584155952,
-79.4916477111548));
#29674=CARTESIAN_POINT('Ctrl Pts',(-5.90570478328609,-30.0007970560453,
-79.4895536575758));
#29675=CARTESIAN_POINT('Ctrl Pts',(-5.90173064346982,-30.0007380879181,
-79.4874294492513));
#29676=CARTESIAN_POINT('Ctrl Pts',(-5.89767668975181,-30.0006815142988,
-79.4852625989908));
#29677=CARTESIAN_POINT('Ctrl Pts',(-5.89333842135675,-30.0006209730194,
-79.4829437816939));
#29678=CARTESIAN_POINT('Ctrl Pts',(-5.88890914683469,-30.000563210484,-79.4805763431629));
#29679=CARTESIAN_POINT('Ctrl Pts',(-5.88441427394656,-30.0005090020521,
-79.4781738543067));
#29680=CARTESIAN_POINT('Ctrl Pts',(-5.87941082856876,-30.0004486602059,
-79.4754995357972));
#29681=CARTESIAN_POINT('Ctrl Pts',(-5.87432672334003,-30.0003927773851,
-79.4727821196766));
#29682=CARTESIAN_POINT('Ctrl Pts',(-5.86925423225277,-30.0003425904324,
-79.4700709150979));
#29683=CARTESIAN_POINT('Ctrl Pts',(-5.86215627755727,-30.0002723636521,
-79.4662771169545));
#29684=CARTESIAN_POINT('Ctrl Pts',(-5.85508269024457,-30.0002135200039,
-79.4624963505019));
#29685=CARTESIAN_POINT('Ctrl Pts',(-5.84838446975869,-30.0001672203483,
-79.458916194205));
#29686=CARTESIAN_POINT('Ctrl Pts',(-5.84284768581393,-30.0001289488119,
-79.4559568183609));
#29687=CARTESIAN_POINT('Ctrl Pts',(-5.83757231667413,-30.0000991731415,
-79.4531371523948));
#29688=CARTESIAN_POINT('Ctrl Pts',(-5.83274900607812,-30.0000766073763,
-79.450559082205));
#29689=CARTESIAN_POINT('Ctrl Pts',(-5.82874247887498,-30.0000578629163,
-79.4484175845466));
#29690=CARTESIAN_POINT('Ctrl Pts',(-5.82504874387763,-30.0000440365559,
-79.4464432539887));
#29691=CARTESIAN_POINT('Ctrl Pts',(-5.82174274620944,-30.0000337677252,
-79.4446761456858));
#29692=CARTESIAN_POINT('Ctrl Pts',(-5.81868753713252,-30.0000242778744,
-79.4430430878712));
#29693=CARTESIAN_POINT('Ctrl Pts',(-5.81596405942472,-30.0000178010199,
-79.4415873205933));
#29694=CARTESIAN_POINT('Ctrl Pts',(-5.81358977837239,-30.0000131915893,
-79.4403181802751));
#29695=CARTESIAN_POINT('Ctrl Pts',(-5.81143204918921,-30.0000090025726,
-79.4391647948748));
#29696=CARTESIAN_POINT('Ctrl Pts',(-5.80956279681059,-30.0000063473931,
-79.4381655849932));
#29697=CARTESIAN_POINT('Ctrl Pts',(-5.80795543373066,-30.000004520639,-79.4373063426729));
#29698=CARTESIAN_POINT('Ctrl Pts',(-5.80640524598471,-30.0000027588642,
-79.436477664366));
#29699=CARTESIAN_POINT('Ctrl Pts',(-5.80509895162393,-30.0000017661867,
-79.4357793357));
#29700=CARTESIAN_POINT('Ctrl Pts',(-5.8039708127979,-30.0000011262397,-79.4351762238893));
#29701=CARTESIAN_POINT('Ctrl Pts',(-5.80289072093286,-30.0000005135478,
-79.4345987983584));
#29702=CARTESIAN_POINT('Ctrl Pts',(-5.80197407678276,-30.0000002263774,
-79.4341087289835));
#29703=CARTESIAN_POINT('Ctrl Pts',(-5.8011210264025,-30.0000000897643,-79.4336526482453));
#29704=CARTESIAN_POINT('Ctrl Pts',(-5.80073919554487,-30.0000000286154,
-79.4334485035623));
#29705=CARTESIAN_POINT('Ctrl Pts',(-5.80036951503659,-30.,-79.4332508528029));
#29706=CARTESIAN_POINT('Ctrl Pts',(-5.8,-30.,-79.4330532904862));
#29707=CARTESIAN_POINT('',(-5.26966991411008,-30.,-79.7165266452431));
#29708=CARTESIAN_POINT('Ctrl Pts',(-12.7960010943682,-36.7634229774484,
-79.559527160348));
#29709=CARTESIAN_POINT('Ctrl Pts',(-12.796112684693,-36.766722900773,-79.5577622689418));
#29710=CARTESIAN_POINT('Ctrl Pts',(-12.7966304463649,-36.779733004731,-79.5508027625369));
#29711=CARTESIAN_POINT('Ctrl Pts',(-12.798503621254,-36.8493462580203,-79.5135787011833));
#29712=CARTESIAN_POINT('Ctrl Pts',(-12.7995831813545,-36.9140618669959,
-79.4789882204304));
#29713=CARTESIAN_POINT('Ctrl Pts',(-12.800077777097,-36.9836467597157,-79.4417959628394));
#29714=CARTESIAN_POINT('Ctrl Pts',(-12.8,-36.9966978147859,-79.4348188136624));
#29715=CARTESIAN_POINT('Ctrl Pts',(-12.8,-37.,-79.4330532904862));
#29716=CARTESIAN_POINT('Ctrl Pts',(-12.7810518328599,-36.9201809478066,
-79.8527909466985));
#29717=CARTESIAN_POINT('Ctrl Pts',(-12.7813470858521,-36.9262391322969,
-79.8495905651427));
#29718=CARTESIAN_POINT('Ctrl Pts',(-12.7831737363863,-36.9560219574473,
-79.8337980696517));
#29719=CARTESIAN_POINT('Ctrl Pts',(-12.7889123048375,-37.0722811924033,
-79.7718566610738));
#29720=CARTESIAN_POINT('Ctrl Pts',(-12.7951961994244,-37.2013837171206,
-79.7031096229565));
#29721=CARTESIAN_POINT('Ctrl Pts',(-12.7992412708901,-37.3176322921036,
-79.6411502857689));
#29722=CARTESIAN_POINT('Ctrl Pts',(-12.8,-37.3474826193307,-79.6252655486096));
#29723=CARTESIAN_POINT('Ctrl Pts',(-12.8,-37.3535533905933,-79.6220355269908));
#29724=CARTESIAN_POINT('Ctrl Pts',(-12.7661025713516,-37.0769389181648,
-80.146054733049));
#29725=CARTESIAN_POINT('Ctrl Pts',(-12.7668146458603,-37.0857693916081,
-80.1414232484696));
#29726=CARTESIAN_POINT('Ctrl Pts',(-12.771474141461,-37.1146188178936,-80.126276652849));
#29727=CARTESIAN_POINT('Ctrl Pts',(-12.7845596965995,-37.3111973977879,
-80.0204512333998));
#29728=CARTESIAN_POINT('Ctrl Pts',(-12.7958833886632,-37.4728678413485,
-79.9346812492863));
#29729=CARTESIAN_POINT('Ctrl Pts',(-12.7990076133253,-37.6692758524317,
-79.8304581598936));
#29730=CARTESIAN_POINT('Ctrl Pts',(-12.8,-37.6982674238754,-79.8157122835568));
#29731=CARTESIAN_POINT('Ctrl Pts',(-12.8,-37.7071067811866,-79.8110177634954));
#29732=CARTESIAN_POINT('Ctrl Pts',(-12.7511533098433,-37.2336968885229,
-80.4393185193995));
#29733=CARTESIAN_POINT('Ctrl Pts',(-12.7525119116407,-37.2452680428387,
-80.4332845365905));
#29734=CARTESIAN_POINT('Ctrl Pts',(-12.7587851319936,-37.2908525231663,
-80.4097062662184));
#29735=CARTESIAN_POINT('Ctrl Pts',(-12.7815887113731,-37.5340742166441,
-80.281832792717));
#29736=CARTESIAN_POINT('Ctrl Pts',(-12.7948941008387,-37.7601548957666,
-80.1608661463623));
#29737=CARTESIAN_POINT('Ctrl Pts',(-12.8009520655495,-38.0032538535837,
-80.0305401854391));
#29738=CARTESIAN_POINT('Ctrl Pts',(-12.8,-38.0490522284202,-80.006159018504));
#29739=CARTESIAN_POINT('Ctrl Pts',(-12.8,-38.0606601717798,-80.));
#29740=CARTESIAN_POINT('',(-12.8,-37.,-79.4330532904862));
#29741=CARTESIAN_POINT('',(-12.7960010943682,-36.7634229774484,-79.559527160348));
#29742=CARTESIAN_POINT('Ctrl Pts',(-12.8,-37.,-79.4330532904862));
#29743=CARTESIAN_POINT('Ctrl Pts',(-12.8,-36.9991700472799,-79.433497027184));
#29744=CARTESIAN_POINT('Ctrl Pts',(-12.7999998681034,-36.9983360052531,
-79.4339429495663));
#29745=CARTESIAN_POINT('Ctrl Pts',(-12.7999995080477,-36.9973756274263,
-79.4344563936114));
#29746=CARTESIAN_POINT('Ctrl Pts',(-12.7999991342866,-36.9963786928142,
-79.4349893819059));
#29747=CARTESIAN_POINT('Ctrl Pts',(-12.7999985165436,-36.9952458083565,
-79.4355950301756));
#29748=CARTESIAN_POINT('Ctrl Pts',(-12.7999973347952,-36.9938915746925,
-79.4363189798575));
#29749=CARTESIAN_POINT('Ctrl Pts',(-12.7999960976967,-36.9924739120601,
-79.4370768375589));
#29750=CARTESIAN_POINT('Ctrl Pts',(-12.7999942436752,-36.9908139133176,
-79.4379642131993));
#29751=CARTESIAN_POINT('Ctrl Pts',(-12.7999911447529,-36.9888656665758,
-79.4390056428451));
#29752=CARTESIAN_POINT('Ctrl Pts',(-12.7999878573614,-36.9867989320079,
-79.4401104098148));
#29753=CARTESIAN_POINT('Ctrl Pts',(-12.7999831623485,-36.9844081334042,
-79.4413883725713));
#29754=CARTESIAN_POINT('Ctrl Pts',(-12.7999760573464,-36.9816916254731,
-79.4428404082825));
#29755=CARTESIAN_POINT('Ctrl Pts',(-12.7999683372862,-36.9787399578497,
-79.4444181422356));
#29756=CARTESIAN_POINT('Ctrl Pts',(-12.7999577493633,-36.9754042150751,
-79.4462011422145));
#29757=CARTESIAN_POINT('Ctrl Pts',(-12.7999429445767,-36.971737433388,-79.4481610614896));
#29758=CARTESIAN_POINT('Ctrl Pts',(-12.7999255589313,-36.9674314364342,
-79.4504626455894));
#29759=CARTESIAN_POINT('Ctrl Pts',(-12.7999022941935,-36.962669730668,-79.4530077769879));
#29760=CARTESIAN_POINT('Ctrl Pts',(-12.7998716028383,-36.957602549858,-79.4557161648616));
#29761=CARTESIAN_POINT('Ctrl Pts',(-12.7998303537853,-36.9507922800498,
-79.4593562268323));
#29762=CARTESIAN_POINT('Ctrl Pts',(-12.7997754571375,-36.9434364114665,
-79.4632878755981));
#29763=CARTESIAN_POINT('Ctrl Pts',(-12.7997070636587,-36.9359607700949,
-79.4672835422778));
#29764=CARTESIAN_POINT('Ctrl Pts',(-12.7996614454932,-36.9309745484407,
-79.4699486353087));
#29765=CARTESIAN_POINT('Ctrl Pts',(-12.7996099514239,-36.9259365295086,
-79.4726414139089));
#29766=CARTESIAN_POINT('Ctrl Pts',(-12.799553634361,-36.9209498911825,-79.4753067403585));
#29767=CARTESIAN_POINT('Ctrl Pts',(-12.7995030421141,-36.9164701611609,
-79.4777011275455));
#29768=CARTESIAN_POINT('Ctrl Pts',(-12.7994485979144,-36.9120324824234,
-79.4800730469208));
#29769=CARTESIAN_POINT('Ctrl Pts',(-12.7993911715046,-36.9076786684244,
-79.4824001575494));
#29770=CARTESIAN_POINT('Ctrl Pts',(-12.7993375275474,-36.9036116231,-79.4845739905159));
#29771=CARTESIAN_POINT('Ctrl Pts',(-12.7992813111153,-36.8996181331004,
-79.4867085227894));
#29772=CARTESIAN_POINT('Ctrl Pts',(-12.7992228531719,-36.8956953901507,
-79.4888052645999));
#29773=CARTESIAN_POINT('Ctrl Pts',(-12.7991663978579,-36.8919070309902,
-79.4908301770519));
#29774=CARTESIAN_POINT('Ctrl Pts',(-12.7991078794155,-36.888185055055,-79.492819629682));
#29775=CARTESIAN_POINT('Ctrl Pts',(-12.7990468226819,-36.8844856116882,
-79.4947970740634));
#29776=CARTESIAN_POINT('Ctrl Pts',(-12.7989837615226,-36.8806647196525,
-79.4968394357754));
#29777=CARTESIAN_POINT('Ctrl Pts',(-12.7989179009539,-36.8768614401243,
-79.4988724221631));
#29778=CARTESIAN_POINT('Ctrl Pts',(-12.7988478958076,-36.8730034199306,
-79.500934726048));
#29779=CARTESIAN_POINT('Ctrl Pts',(-12.7987768114531,-36.869085924007,-79.5030288226719));
#29780=CARTESIAN_POINT('Ctrl Pts',(-12.7987014293895,-36.8651121239306,
-79.5051530744746));
#29781=CARTESIAN_POINT('Ctrl Pts',(-12.798620957786,-36.861058684193,-79.507319968484));
#29782=CARTESIAN_POINT('Ctrl Pts',(-12.7985348425268,-36.8567209675521,
-79.5096388316748));
#29783=CARTESIAN_POINT('Ctrl Pts',(-12.7984428756104,-36.8522924453854,
-79.5120063163369));
#29784=CARTESIAN_POINT('Ctrl Pts',(-12.7983451408915,-36.8477985251063,
-79.5144088487625));
#29785=CARTESIAN_POINT('Ctrl Pts',(-12.7982363480041,-36.8427961414171,
-79.517083215078));
#29786=CARTESIAN_POINT('Ctrl Pts',(-12.7981203741976,-36.8377133475194,
-79.5198006757509));
#29787=CARTESIAN_POINT('Ctrl Pts',(-12.7979991018748,-36.8326423884013,
-79.5225119154));
#29788=CARTESIAN_POINT('Ctrl Pts',(-12.7978294071761,-36.8255466648324,
-79.5263057158687));
#29789=CARTESIAN_POINT('Ctrl Pts',(-12.797649162788,-36.8184757467536,-79.5300864660878));
#29790=CARTESIAN_POINT('Ctrl Pts',(-12.7974690699909,-36.8117804087757,
-79.5336665753703));
#29791=CARTESIAN_POINT('Ctrl Pts',(-12.797320200581,-36.8062458675276,-79.5366259872121));
#29792=CARTESIAN_POINT('Ctrl Pts',(-12.7971716766398,-36.8009728944587,
-79.5394456609008));
#29793=CARTESIAN_POINT('Ctrl Pts',(-12.7970312260022,-36.7961519626054,
-79.5420236982032));
#29794=CARTESIAN_POINT('Ctrl Pts',(-12.7969145602557,-36.7921474409935,
-79.5441651526787));
#29795=CARTESIAN_POINT('Ctrl Pts',(-12.7968035511635,-36.7884556925945,
-79.5461394144843));
#29796=CARTESIAN_POINT('Ctrl Pts',(-12.7967020909069,-36.7851515624929,
-79.5479064262232));
#29797=CARTESIAN_POINT('Ctrl Pts',(-12.7966083305111,-36.78209818419,-79.5495393387112));
#29798=CARTESIAN_POINT('Ctrl Pts',(-12.7965227697646,-36.7793764113463,
-79.5509949492069));
#29799=CARTESIAN_POINT('Ctrl Pts',(-12.7964471432921,-36.7770036522266,
-79.5522639237828));
#29800=CARTESIAN_POINT('Ctrl Pts',(-12.7963784121474,-36.7748472320619,
-79.5534171981886));
#29801=CARTESIAN_POINT('Ctrl Pts',(-12.7963178972973,-36.7729791573364,
-79.5544162789617));
#29802=CARTESIAN_POINT('Ctrl Pts',(-12.7962654049679,-36.7713728291545,
-79.5552753781006));
#29803=CARTESIAN_POINT('Ctrl Pts',(-12.7962147798707,-36.7698236405127,
-79.5561039177746));
#29804=CARTESIAN_POINT('Ctrl Pts',(-12.7961716284115,-36.7685182119286,
-79.5568020948707));
#29805=CARTESIAN_POINT('Ctrl Pts',(-12.7961341448816,-36.7673908281644,
-79.5574050490616));
#29806=CARTESIAN_POINT('Ctrl Pts',(-12.7960982577448,-36.7663114587615,
-79.5579823239218));
#29807=CARTESIAN_POINT('Ctrl Pts',(-12.7960675687105,-36.7653954357194,
-79.5584722369981));
#29808=CARTESIAN_POINT('Ctrl Pts',(-12.7960388778786,-36.7645429567618,
-79.5589281651919));
#29809=CARTESIAN_POINT('Ctrl Pts',(-12.7960260391719,-36.7641614855156,
-79.5591321860592));
#29810=CARTESIAN_POINT('Ctrl Pts',(-12.7960135782664,-36.7637921484035,
-79.5593297173829));
#29811=CARTESIAN_POINT('Ctrl Pts',(-12.7960010943682,-36.7634229774484,
-79.559527160348));
#29812=CARTESIAN_POINT('',(-12.7511533098433,-37.2336968885229,-80.4393185193995));
#29813=CARTESIAN_POINT('Ctrl Pts',(-12.7511533098433,-37.2336968885229,
-80.4393185193995));
#29814=CARTESIAN_POINT('Ctrl Pts',(-12.7661025713516,-37.0769389181648,
-80.146054733049));
#29815=CARTESIAN_POINT('Ctrl Pts',(-12.7810518328599,-36.9201809478066,
-79.8527909466985));
#29816=CARTESIAN_POINT('Ctrl Pts',(-12.7960010943682,-36.7634229774484,
-79.559527160348));
#29817=CARTESIAN_POINT('',(-12.8,-38.0606601717798,-80.));
#29818=CARTESIAN_POINT('Ctrl Pts',(-12.7511533098433,-37.2336968885229,
-80.4393185193995));
#29819=CARTESIAN_POINT('Ctrl Pts',(-12.7513994405692,-37.2357931735541,
-80.4382253745416));
#29820=CARTESIAN_POINT('Ctrl Pts',(-12.7516451610574,-37.2378933689947,
-80.4371300040475));
#29821=CARTESIAN_POINT('Ctrl Pts',(-12.7519098980542,-37.2401660578997,
-80.4359446637797));
#29822=CARTESIAN_POINT('Ctrl Pts',(-12.7521813734055,-37.2424965935867,
-80.4347291530298));
#29823=CARTESIAN_POINT('Ctrl Pts',(-12.7524728330613,-37.2450083893932,
-80.4334190997504));
#29824=CARTESIAN_POINT('Ctrl Pts',(-12.7527989349955,-37.24783495635,-80.4319448106882));
#29825=CARTESIAN_POINT('Ctrl Pts',(-12.7531345289436,-37.2507437976206,
-80.4304276087488));
#29826=CARTESIAN_POINT('Ctrl Pts',(-12.7535068003015,-37.2539858554197,
-80.42873654726));
#29827=CARTESIAN_POINT('Ctrl Pts',(-12.7539253120768,-37.2576582073246,
-80.426820658855));
#29828=CARTESIAN_POINT('Ctrl Pts',(-12.7543667487184,-37.2615317200594,
-80.4247998236171));
#29829=CARTESIAN_POINT('Ctrl Pts',(-12.7548596320871,-37.2658839386598,
-80.4225288661114));
#29830=CARTESIAN_POINT('Ctrl Pts',(-12.755408172194,-37.2707766668765,-80.4199748565295));
#29831=CARTESIAN_POINT('Ctrl Pts',(-12.7559812991956,-37.275888699009,-80.4173063700591));
#29832=CARTESIAN_POINT('Ctrl Pts',(-12.7566151458086,-37.2815905684644,
-80.4143289939935));
#29833=CARTESIAN_POINT('Ctrl Pts',(-12.7573073447791,-37.2878992679656,
-80.411032794402));
#29834=CARTESIAN_POINT('Ctrl Pts',(-12.7580393314685,-37.2945705926274,
-80.4075471286764));
#29835=CARTESIAN_POINT('Ctrl Pts',(-12.7588364999907,-37.30192023826,-80.4037050658652));
#29836=CARTESIAN_POINT('Ctrl Pts',(-12.7596890377365,-37.3099134194748,
-80.3995233101776));
#29837=CARTESIAN_POINT('Ctrl Pts',(-12.7606097179899,-37.3185454878402,
-80.395007310851));
#29838=CARTESIAN_POINT('Ctrl Pts',(-12.7615948440084,-37.3279276832095,
-80.3900953298116));
#29839=CARTESIAN_POINT('Ctrl Pts',(-12.7626256502735,-37.3379589184685,
-80.3848383516342));
#29840=CARTESIAN_POINT('Ctrl Pts',(-12.7637911119095,-37.3493005451655,
-80.3788946485406));
#29841=CARTESIAN_POINT('Ctrl Pts',(-12.7650147097049,-37.3614711578117,
-80.3725102492067));
#29842=CARTESIAN_POINT('Ctrl Pts',(-12.7662645085333,-37.3742620271656,
-80.3657921301537));
#29843=CARTESIAN_POINT('Ctrl Pts',(-12.7681310603188,-37.3933649575649,
-80.3557587417162));
#29844=CARTESIAN_POINT('Ctrl Pts',(-12.7700542611625,-37.4138480222161,
-80.3449824308113));
#29845=CARTESIAN_POINT('Ctrl Pts',(-12.771933161456,-37.4348978198511,-80.3338856192622));
#29846=CARTESIAN_POINT('Ctrl Pts',(-12.7732621154593,-37.4497864293912,
-80.3260367982351));
#29847=CARTESIAN_POINT('Ctrl Pts',(-12.7745690686291,-37.4649546500062,
-80.3180298208842));
#29848=CARTESIAN_POINT('Ctrl Pts',(-12.7758280668251,-37.4801342690844,
-80.3100055650248));
#29849=CARTESIAN_POINT('Ctrl Pts',(-12.7768947488483,-37.4929951507302,
-80.3032070410057));
#29850=CARTESIAN_POINT('Ctrl Pts',(-12.7779271339726,-37.5058636123494,
-80.2963964675831));
#29851=CARTESIAN_POINT('Ctrl Pts',(-12.7789158806655,-37.518612876001,-80.2896410489724));
#29852=CARTESIAN_POINT('Ctrl Pts',(-12.7798229044688,-37.5303083746442,
-80.2834439860397));
#29853=CARTESIAN_POINT('Ctrl Pts',(-12.780693275662,-37.5419031904326,-80.2772935520739));
#29854=CARTESIAN_POINT('Ctrl Pts',(-12.7815244506041,-37.5533390685944,
-80.2712210383768));
#29855=CARTESIAN_POINT('Ctrl Pts',(-12.7823077096733,-37.5641156871265,
-80.2654985951398));
#29856=CARTESIAN_POINT('Ctrl Pts',(-12.7830562158113,-37.574750894505,-80.2598455004758));
#29857=CARTESIAN_POINT('Ctrl Pts',(-12.7837713234296,-37.5852372054239,
-80.2542662705478));
#29858=CARTESIAN_POINT('Ctrl Pts',(-12.7844546559708,-37.5952575678206,
-80.2489349480068));
#29859=CARTESIAN_POINT('Ctrl Pts',(-12.7851075373859,-37.6051417606873,
-80.2436711904462));
#29860=CARTESIAN_POINT('Ctrl Pts',(-12.785733730508,-37.6149255321358,-80.2384566030175));
#29861=CARTESIAN_POINT('Ctrl Pts',(-12.7863647839694,-37.6247852425343,
-80.2332015413918));
#29862=CARTESIAN_POINT('Ctrl Pts',(-12.7869687646608,-37.6345423851848,
-80.2279967299011));
#29863=CARTESIAN_POINT('Ctrl Pts',(-12.7875516726604,-37.6442838772853,
-80.2227966528135));
#29864=CARTESIAN_POINT('Ctrl Pts',(-12.7881141164258,-37.6536833734367,
-80.2177791355722));
#29865=CARTESIAN_POINT('Ctrl Pts',(-12.7886574186774,-37.6630762514784,
-80.2127618146277));
#29866=CARTESIAN_POINT('Ctrl Pts',(-12.7891861182228,-37.6725507961374,
-80.2076983078163));
#29867=CARTESIAN_POINT('Ctrl Pts',(-12.7897476952908,-37.6826145214739,
-80.2023199235641));
#29868=CARTESIAN_POINT('Ctrl Pts',(-12.7902927397347,-37.692770424443,-80.1968894029537));
#29869=CARTESIAN_POINT('Ctrl Pts',(-12.7908223045103,-37.7030685797929,
-80.1913806465253));
#29870=CARTESIAN_POINT('Ctrl Pts',(-12.791368938445,-37.7136986697069,-80.1856943294948));
#29871=CARTESIAN_POINT('Ctrl Pts',(-12.7918989840159,-37.7244799526093,
-80.1799248452));
#29872=CARTESIAN_POINT('Ctrl Pts',(-12.7924102981559,-37.735413051101,-80.1740724096529));
#29873=CARTESIAN_POINT('Ctrl Pts',(-12.792952958374,-37.7470164024437,-80.1678611909471));
#29874=CARTESIAN_POINT('Ctrl Pts',(-12.793474411486,-37.7587904314581,-80.1615567035672));
#29875=CARTESIAN_POINT('Ctrl Pts',(-12.7939700304283,-37.770680649105,-80.1551886521419));
#29876=CARTESIAN_POINT('Ctrl Pts',(-12.7945089628702,-37.7836099855033,
-80.1482640792262));
#29877=CARTESIAN_POINT('Ctrl Pts',(-12.7950171958874,-37.7966762206018,
-80.141264600033));
#29878=CARTESIAN_POINT('Ctrl Pts',(-12.7954885347944,-37.8097519144859,
-80.1342591058519));
#29879=CARTESIAN_POINT('Ctrl Pts',(-12.7960391658972,-37.8250273004919,
-80.1260750944542));
#29880=CARTESIAN_POINT('Ctrl Pts',(-12.7965391522779,-37.8403147035479,
-80.1178833489533));
#29881=CARTESIAN_POINT('Ctrl Pts',(-12.7969821268525,-37.8553453477091,
-80.1098288897853));
#29882=CARTESIAN_POINT('Ctrl Pts',(-12.7975461188403,-37.8744822538933,
-80.0995740112976));
#29883=CARTESIAN_POINT('Ctrl Pts',(-12.7980169429444,-37.8931974999971,
-80.0895446215398));
#29884=CARTESIAN_POINT('Ctrl Pts',(-12.7983966214117,-37.9108833519335,
-80.0800683678505));
#29885=CARTESIAN_POINT('Ctrl Pts',(-12.7986667701735,-37.9234671864481,
-80.0733258253554));
#29886=CARTESIAN_POINT('Ctrl Pts',(-12.7988912189896,-37.9355281057759,
-80.0668642654862));
#29887=CARTESIAN_POINT('Ctrl Pts',(-12.7990759418347,-37.9468694211329,
-80.0607896272218));
#29888=CARTESIAN_POINT('Ctrl Pts',(-12.7992418553829,-37.9570559136128,
-80.0553335354853));
#29889=CARTESIAN_POINT('Ctrl Pts',(-12.7993758428282,-37.9666612296763,
-80.0501899332581));
#29890=CARTESIAN_POINT('Ctrl Pts',(-12.7994842519168,-37.9755767510305,
-80.0454172471301));
#29891=CARTESIAN_POINT('Ctrl Pts',(-12.7995855041482,-37.9839036952367,
-80.0409596400511));
#29892=CARTESIAN_POINT('Ctrl Pts',(-12.7996645158678,-37.9916285000599,
-80.0368258127267));
#29893=CARTESIAN_POINT('Ctrl Pts',(-12.7997270277937,-37.9987011336137,
-80.0330426135706));
#29894=CARTESIAN_POINT('Ctrl Pts',(-12.7997864674487,-38.0054261687645,
-80.0294453471332));
#29895=CARTESIAN_POINT('Ctrl Pts',(-12.799831031352,-38.0115612592219,-80.0261652513481));
#29896=CARTESIAN_POINT('Ctrl Pts',(-12.7998653971875,-38.0171044476453,
-80.0232033000281));
#29897=CARTESIAN_POINT('Ctrl Pts',(-12.7999000951572,-38.0227012091317,
-80.0202127224387));
#29898=CARTESIAN_POINT('Ctrl Pts',(-12.7999244270517,-38.0276938621132,
-80.0175468476837));
#29899=CARTESIAN_POINT('Ctrl Pts',(-12.7999423966669,-38.0321313874579,
-80.0151792626433));
#29900=CARTESIAN_POINT('Ctrl Pts',(-12.7999586895953,-38.0361548616677,
-80.013032589304));
#29901=CARTESIAN_POINT('Ctrl Pts',(-12.7999697470036,-38.0397222527165,
-80.0111309840731));
#29902=CARTESIAN_POINT('Ctrl Pts',(-12.7999777607813,-38.0429130718287,
-80.0094316690052));
#29903=CARTESIAN_POINT('Ctrl Pts',(-12.799985593692,-38.0460318757299,-80.0077707066388));
#29904=CARTESIAN_POINT('Ctrl Pts',(-12.79999051485,-38.0487907196809,-80.006303109571));
#29905=CARTESIAN_POINT('Ctrl Pts',(-12.7999938354508,-38.0513071548013,
-80.0049656981994));
#29906=CARTESIAN_POINT('Ctrl Pts',(-12.7999970603764,-38.0537510847359,
-80.003666821205));
#29907=CARTESIAN_POINT('Ctrl Pts',(-12.7999987706598,-38.0559662730045,
-80.0024907892758));
#29908=CARTESIAN_POINT('Ctrl Pts',(-12.7999995399946,-38.0581037631129,
-80.0013564738542));
#29909=CARTESIAN_POINT('Ctrl Pts',(-12.7999998496093,-38.0589639847485,
-80.0008999745874));
#29910=CARTESIAN_POINT('Ctrl Pts',(-12.8,-38.059812131143,-80.0004499589473));
#29911=CARTESIAN_POINT('Ctrl Pts',(-12.8,-38.0606601717798,-80.));
#29912=CARTESIAN_POINT('',(-12.8,-37.5303300858899,-79.7165266452431));
#29913=CARTESIAN_POINT('Ctrl Pts',(-12.7511533098433,-37.2336968885229,
-80.4393185193995));
#29914=CARTESIAN_POINT('Ctrl Pts',(-12.6502151549565,-36.3740108725136,
-80.8876169778077));
#29915=CARTESIAN_POINT('Ctrl Pts',(-12.1730890667104,-34.7673104933084,
-81.6648966847297));
#29916=CARTESIAN_POINT('Ctrl Pts',(-11.2444873881411,-33.3688875479671,
-82.0000000010328));
#29917=CARTESIAN_POINT('Ctrl Pts',(-10.7999999953529,-32.8445654686786,
-82.));
#29918=CARTESIAN_POINT('Ctrl Pts',(-12.7661025713516,-37.0769389181648,
-80.146054733049));
#29919=CARTESIAN_POINT('Ctrl Pts',(-12.6891256583696,-36.2174179501799,
-80.5980934851221));
#29920=CARTESIAN_POINT('Ctrl Pts',(-12.254521024505,-34.617670241717,-81.4026172457878));
#29921=CARTESIAN_POINT('Ctrl Pts',(-11.3507989284016,-33.237189874179,-81.7954256760992));
#29922=CARTESIAN_POINT('Ctrl Pts',(-10.9136110332455,-32.7213815205079,
-81.8224303038976));
#29923=CARTESIAN_POINT('Ctrl Pts',(-12.7810518328599,-36.9201809478066,
-79.8527909466985));
#29924=CARTESIAN_POINT('Ctrl Pts',(-12.7280361617827,-36.0608250278462,
-80.3085699924365));
#29925=CARTESIAN_POINT('Ctrl Pts',(-12.3359529822995,-34.4680299901255,
-81.1403378068459));
#29926=CARTESIAN_POINT('Ctrl Pts',(-11.4571104686622,-33.105492200391,-81.5908513511656));
#29927=CARTESIAN_POINT('Ctrl Pts',(-11.0272220711382,-32.5981975723372,
-81.6448606077953));
#29928=CARTESIAN_POINT('Ctrl Pts',(-12.7960010943682,-36.7634229774484,
-79.559527160348));
#29929=CARTESIAN_POINT('Ctrl Pts',(-12.7669466651958,-35.9042321055125,
-80.0190464997509));
#29930=CARTESIAN_POINT('Ctrl Pts',(-12.4173849400941,-34.3183897385341,
-80.878058367904));
#29931=CARTESIAN_POINT('Ctrl Pts',(-11.5634220089227,-32.973794526603,-81.386277026232));
#29932=CARTESIAN_POINT('Ctrl Pts',(-11.1408331090309,-32.4750136241665,
-81.467290911693));
#29933=CARTESIAN_POINT('',(-11.1408331090314,-32.4750136241671,-81.4672909116929));
#29934=CARTESIAN_POINT('Ctrl Pts',(-12.7960010943682,-36.7634229774484,
-79.559527160348));
#29935=CARTESIAN_POINT('Ctrl Pts',(-12.7669466651958,-35.9042321055125,
-80.0190464997509));
#29936=CARTESIAN_POINT('Ctrl Pts',(-12.4173849400941,-34.3183897385341,
-80.878058367904));
#29937=CARTESIAN_POINT('Ctrl Pts',(-11.5634220089227,-32.973794526603,-81.386277026232));
#29938=CARTESIAN_POINT('Ctrl Pts',(-11.1408331090309,-32.4750136241665,
-81.467290911693));
#29939=CARTESIAN_POINT('',(-10.7999999970626,-32.8445654672303,-82.));
#29940=CARTESIAN_POINT('',(-11.1408331090314,-32.4750136241671,-81.4672909116929));
#29941=CARTESIAN_POINT('Ctrl Pts',(-10.7999999953529,-32.8445654686786,
-82.));
#29942=CARTESIAN_POINT('Ctrl Pts',(-11.2444873881411,-33.3688875479671,
-82.0000000010328));
#29943=CARTESIAN_POINT('Ctrl Pts',(-12.1730890667104,-34.7673104933084,
-81.6648966847297));
#29944=CARTESIAN_POINT('Ctrl Pts',(-12.6502151549565,-36.3740108725136,
-80.8876169778077));
#29945=CARTESIAN_POINT('Ctrl Pts',(-12.7511533098433,-37.2336968885229,
-80.4393185193995));
#29946=CARTESIAN_POINT('Origin',(-5.79999999999999,-37.,-81.75));
#29947=CARTESIAN_POINT('',(-10.4428571428571,-32.4509476205455,-82.));
#29948=CARTESIAN_POINT('',(-10.8,-32.1010205144336,-81.5));
#29949=CARTESIAN_POINT('',(-10.4428571428571,-32.4509476205455,-82.));
#29950=CARTESIAN_POINT('',(-10.6989794855664,-32.,-81.5));
#29951=CARTESIAN_POINT('Origin',(-5.79999999999999,-37.,-81.5));
#29952=CARTESIAN_POINT('',(-10.3490523794545,-32.3571428571429,-82.));
#29953=CARTESIAN_POINT('',(-10.6989794855664,-32.,-81.5));
#29954=CARTESIAN_POINT('Origin',(-5.79999999999999,-37.,-82.));
#29955=CARTESIAN_POINT('Ctrl Pts',(-10.7999999953534,-32.8445654686792,
-82.));
#29956=CARTESIAN_POINT('Ctrl Pts',(-10.6842569540723,-32.7080337400726,
-82.));
#29957=CARTESIAN_POINT('Ctrl Pts',(-10.5665688864269,-32.5772103901022,
-82.));
#29958=CARTESIAN_POINT('Ctrl Pts',(-10.4428571428571,-32.4509476205455,
-82.));
#29959=CARTESIAN_POINT('Ctrl Pts',(-10.9136110332461,-32.7213815205085,
-81.8224303038976));
#29960=CARTESIAN_POINT('Ctrl Pts',(-10.7997687569007,-32.5870667377815,
-81.8294622194963));
#29961=CARTESIAN_POINT('Ctrl Pts',(-10.6833507226253,-32.4582555164613,
-81.8333333333333));
#29962=CARTESIAN_POINT('Ctrl Pts',(-10.5619047619048,-32.3343052518416,
-81.8333333333333));
#29963=CARTESIAN_POINT('Ctrl Pts',(-11.0272220711388,-32.5981975723378,
-81.6448606077953));
#29964=CARTESIAN_POINT('Ctrl Pts',(-10.9152805597292,-32.4660997354905,
-81.6589244389925));
#29965=CARTESIAN_POINT('Ctrl Pts',(-10.8001325588236,-32.3393006428204,
-81.6666666666667));
#29966=CARTESIAN_POINT('Ctrl Pts',(-10.6809523809524,-32.2176628831376,
-81.6666666666667));
#29967=CARTESIAN_POINT('Ctrl Pts',(-11.1408331090314,-32.4750136241671,
-81.4672909116929));
#29968=CARTESIAN_POINT('Ctrl Pts',(-11.0307923625576,-32.3451327331994,
-81.4883866584888));
#29969=CARTESIAN_POINT('Ctrl Pts',(-10.916914395022,-32.2203457691795,-81.5));
#29970=CARTESIAN_POINT('Ctrl Pts',(-10.8,-32.1010205144336,-81.5));
#29971=CARTESIAN_POINT('Ctrl Pts',(-10.4428571428571,-32.4509476205455,
-82.));
#29972=CARTESIAN_POINT('Ctrl Pts',(-10.5665688864269,-32.5772103901022,
-82.));
#29973=CARTESIAN_POINT('Ctrl Pts',(-10.6842569540723,-32.7080337400726,
-82.));
#29974=CARTESIAN_POINT('Ctrl Pts',(-10.7999999953534,-32.8445654686792,
-82.));
#29975=CARTESIAN_POINT('Ctrl Pts',(-11.1408331090314,-32.4750136241671,
-81.4672909116929));
#29976=CARTESIAN_POINT('Ctrl Pts',(-11.0307923625576,-32.3451327331994,
-81.4883866584888));
#29977=CARTESIAN_POINT('Ctrl Pts',(-10.916914395022,-32.2203457691795,-81.5));
#29978=CARTESIAN_POINT('Ctrl Pts',(-10.8,-32.1010205144336,-81.5));
#29979=CARTESIAN_POINT('Ctrl Pts',(-9.95543453132142,-32.0000000046471,
-82.));
#29980=CARTESIAN_POINT('Ctrl Pts',(-9.25633811784897,-31.4073498867012,
-82.000000001377));
#29981=CARTESIAN_POINT('Ctrl Pts',(-7.79517610804797,-30.5212430753724,
-81.5542555113626));
#29982=CARTESIAN_POINT('Ctrl Pts',(-6.21107604659501,-30.124551119002,-80.7755468086672));
#29983=CARTESIAN_POINT('Ctrl Pts',(-5.56630111765684,-30.048846456053,-80.4393174796692));
#29984=CARTESIAN_POINT('Ctrl Pts',(-10.0786184794921,-31.8863889667545,
-81.8224303038976));
#29985=CARTESIAN_POINT('Ctrl Pts',(-9.39087370517329,-31.3034715166025,
-81.7864241176491));
#29986=CARTESIAN_POINT('Ctrl Pts',(-7.94673543863312,-30.4455217633812,
-81.2853561028645));
#29987=CARTESIAN_POINT('Ctrl Pts',(-6.36770343773579,-30.0916304595765,
-80.4850846324629));
#29988=CARTESIAN_POINT('Ctrl Pts',(-5.72305909304156,-30.033897250275,-80.1460536871276));
#29989=CARTESIAN_POINT('Ctrl Pts',(-10.2018024276628,-31.7727779288618,
-81.6448606077953));
#29990=CARTESIAN_POINT('Ctrl Pts',(-9.52540929249762,-31.1995931465039,
-81.5728482339212));
#29991=CARTESIAN_POINT('Ctrl Pts',(-8.09829476921827,-30.36980045139,-81.0164566943663));
#29992=CARTESIAN_POINT('Ctrl Pts',(-6.52433082887656,-30.058709800151,-80.1946224562586));
#29993=CARTESIAN_POINT('Ctrl Pts',(-5.87981706842629,-30.018948044497,-79.8527898945859));
#29994=CARTESIAN_POINT('Ctrl Pts',(-10.3249863758336,-31.6591668909691,
-81.467290911693));
#29995=CARTESIAN_POINT('Ctrl Pts',(-9.65994487982194,-31.0957147764052,
-81.3592723501933));
#29996=CARTESIAN_POINT('Ctrl Pts',(-8.24985409980341,-30.2940791393988,
-80.7475572858682));
#29997=CARTESIAN_POINT('Ctrl Pts',(-6.68095822001734,-30.0257891407254,
-79.9041602800544));
#29998=CARTESIAN_POINT('Ctrl Pts',(-6.03657504381102,-30.0039988387189,
-79.5595261020443));
#29999=CARTESIAN_POINT('',(-9.95543453276968,-32.0000000029374,-82.));
#30000=CARTESIAN_POINT('Ctrl Pts',(-5.56630111765684,-30.048846456053,-80.4393174796692));
#30001=CARTESIAN_POINT('Ctrl Pts',(-6.21107604659501,-30.124551119002,-80.7755468086672));
#30002=CARTESIAN_POINT('Ctrl Pts',(-7.79517610804797,-30.5212430753724,
-81.5542555113626));
#30003=CARTESIAN_POINT('Ctrl Pts',(-9.25633811784897,-31.4073498867012,
-82.000000001377));
#30004=CARTESIAN_POINT('Ctrl Pts',(-9.95543453132142,-32.0000000046471,
-82.));
#30005=CARTESIAN_POINT('',(-10.3249863758329,-31.6591668909686,-81.4672909116929));
#30006=CARTESIAN_POINT('',(-9.95543453276968,-32.0000000029374,-82.));
#30007=CARTESIAN_POINT('Ctrl Pts',(-10.3249863758336,-31.6591668909691,
-81.467290911693));
#30008=CARTESIAN_POINT('Ctrl Pts',(-9.65994487982194,-31.0957147764052,
-81.3592723501933));
#30009=CARTESIAN_POINT('Ctrl Pts',(-8.24985409980341,-30.2940791393988,
-80.7475572858682));
#30010=CARTESIAN_POINT('Ctrl Pts',(-6.68095822001734,-30.0257891407254,
-79.9041602800544));
#30011=CARTESIAN_POINT('Ctrl Pts',(-6.03657504381102,-30.0039988387189,
-79.5595261020443));
#30012=CARTESIAN_POINT('Ctrl Pts',(-10.3490523794545,-32.3571428571429,
-82.));
#30013=CARTESIAN_POINT('Ctrl Pts',(-10.2227896098978,-32.2334311135731,
-82.));
#30014=CARTESIAN_POINT('Ctrl Pts',(-10.0919662599274,-32.1157430459277,
-82.));
#30015=CARTESIAN_POINT('Ctrl Pts',(-9.95543453132077,-32.0000000046466,
-82.));
#30016=CARTESIAN_POINT('Ctrl Pts',(-10.4656947481584,-32.2380952380952,
-81.8333333333333));
#30017=CARTESIAN_POINT('Ctrl Pts',(-10.3417444835387,-32.1166492773747,
-81.8333333333333));
#30018=CARTESIAN_POINT('Ctrl Pts',(-10.2129332622185,-32.0002312430993,
-81.8294622194963));
#30019=CARTESIAN_POINT('Ctrl Pts',(-10.0786184794915,-31.8863889667539,
-81.8224303038976));
#30020=CARTESIAN_POINT('Ctrl Pts',(-10.5823371168624,-32.1190476190476,
-81.6666666666667));
#30021=CARTESIAN_POINT('Ctrl Pts',(-10.4606993571796,-31.9998674411764,
-81.6666666666667));
#30022=CARTESIAN_POINT('Ctrl Pts',(-10.3339002645095,-31.8847194402708,
-81.6589244389925));
#30023=CARTESIAN_POINT('Ctrl Pts',(-10.2018024276622,-31.7727779288612,
-81.6448606077953));
#30024=CARTESIAN_POINT('Ctrl Pts',(-10.6989794855664,-32.,-81.5));
#30025=CARTESIAN_POINT('Ctrl Pts',(-10.5796542308205,-31.883085604978,-81.5));
#30026=CARTESIAN_POINT('Ctrl Pts',(-10.4548672668006,-31.7692076374424,
-81.4883866584888));
#30027=CARTESIAN_POINT('Ctrl Pts',(-10.3249863758329,-31.6591668909686,
-81.4672909116929));
#30028=CARTESIAN_POINT('Ctrl Pts',(-9.95543453132077,-32.0000000046466,
-82.));
#30029=CARTESIAN_POINT('Ctrl Pts',(-10.0919662599274,-32.1157430459277,
-82.));
#30030=CARTESIAN_POINT('Ctrl Pts',(-10.2227896098978,-32.2334311135731,
-82.));
#30031=CARTESIAN_POINT('Ctrl Pts',(-10.3490523794545,-32.3571428571429,
-82.));
#30032=CARTESIAN_POINT('Ctrl Pts',(-10.6989794855664,-32.,-81.5));
#30033=CARTESIAN_POINT('Ctrl Pts',(-10.5796542308205,-31.883085604978,-81.5));
#30034=CARTESIAN_POINT('Ctrl Pts',(-10.4548672668006,-31.7692076374424,
-81.4883866584888));
#30035=CARTESIAN_POINT('Ctrl Pts',(-10.3249863758329,-31.6591668909686,
-81.4672909116929));
#30036=CARTESIAN_POINT('Origin',(25.7,-32.,-80.));
#30037=CARTESIAN_POINT('',(35.1393398282202,-30.,-80.));
#30038=CARTESIAN_POINT('',(25.7,-30.,-80.));
#30039=CARTESIAN_POINT('',(35.9663031078275,-30.0488466897261,-80.4393185174872));
#30040=CARTESIAN_POINT('Ctrl Pts',(35.9663031078275,-30.0488466897261,-80.4393185174872));
#30041=CARTESIAN_POINT('Ctrl Pts',(35.9642068228121,-30.0486005589982,-80.4382253726154));
#30042=CARTESIAN_POINT('Ctrl Pts',(35.9621066273875,-30.048354838508,-80.437130002107));
#30043=CARTESIAN_POINT('Ctrl Pts',(35.9598339385104,-30.0480901015045,-80.4359446618037));
#30044=CARTESIAN_POINT('Ctrl Pts',(35.957503402852,-30.0478186261464,-80.4347291510173));
#30045=CARTESIAN_POINT('Ctrl Pts',(35.9549916070864,-30.0475271664789,-80.4334190976791));
#30046=CARTESIAN_POINT('Ctrl Pts',(35.9521650401915,-30.0472010645251,-80.4319448085208));
#30047=CARTESIAN_POINT('Ctrl Pts',(35.9492561989846,-30.0468654705568,-80.4304276064823));
#30048=CARTESIAN_POINT('Ctrl Pts',(35.9460141412712,-30.0464931991705,-80.4287365448548));
#30049=CARTESIAN_POINT('Ctrl Pts',(35.9423417894798,-30.0460746873567,-80.426820656262));
#30050=CARTESIAN_POINT('Ctrl Pts',(35.9384682768646,-30.0456332506747,-80.424799820826));
#30051=CARTESIAN_POINT('Ctrl Pts',(35.9341160584144,-30.0451403672545,-80.4225288630673));
#30052=CARTESIAN_POINT('Ctrl Pts',(35.929223330381,-30.0445918270853,-80.419974853174));
#30053=CARTESIAN_POINT('Ctrl Pts',(35.9241112984395,-30.0440187000186,-80.4173063663779));
#30054=CARTESIAN_POINT('Ctrl Pts',(35.9184094292111,-30.0433848533287,-80.414328989923));
#30055=CARTESIAN_POINT('Ctrl Pts',(35.9121007299712,-30.0426926542716,-80.4110327898815));
#30056=CARTESIAN_POINT('Ctrl Pts',(35.9054294055848,-30.0419606674906,-80.4075471236796));
#30057=CARTESIAN_POINT('Ctrl Pts',(35.8980797602659,-30.041163498866,-80.4037050603245));
#30058=CARTESIAN_POINT('Ctrl Pts',(35.8900865793965,-30.0403109610116,-80.399523304037));
#30059=CARTESIAN_POINT('Ctrl Pts',(35.8814545114029,-30.0393902806408,-80.3950073040619));
#30060=CARTESIAN_POINT('Ctrl Pts',(35.8720723164423,-30.0384051544974,-80.3900953223086));
#30061=CARTESIAN_POINT('Ctrl Pts',(35.8620410816167,-30.037374348107,-80.384838343375));
#30062=CARTESIAN_POINT('Ctrl Pts',(35.8506994554101,-30.0362088863294,-80.3788946394264));
#30063=CARTESIAN_POINT('Ctrl Pts',(35.8385288432859,-30.0349852883917,-80.3725102391835));
#30064=CARTESIAN_POINT('Ctrl Pts',(35.8257379744632,-30.0337354894307,-80.3657921192093));
#30065=CARTESIAN_POINT('Ctrl Pts',(35.80663504561,-30.0318689375205,-80.3557587297912));
#30066=CARTESIAN_POINT('Ctrl Pts',(35.7861519826339,-30.0299457365785,-80.3449824179376));
#30067=CARTESIAN_POINT('Ctrl Pts',(35.7651021866241,-30.0280668362265,-80.3338856055751));
#30068=CARTESIAN_POINT('Ctrl Pts',(35.7502135775262,-30.0267378821187,-80.3260367835997));
#30069=CARTESIAN_POINT('Ctrl Pts',(35.7350453573012,-30.0254309288662,-80.3180298053536));
#30070=CARTESIAN_POINT('Ctrl Pts',(35.7198657385427,-30.0241719306146,-80.3100055487063));
#30071=CARTESIAN_POINT('Ctrl Pts',(35.7070048572268,-30.0231052485491,-80.303207024051));
#30072=CARTESIAN_POINT('Ctrl Pts',(35.6941363958872,-30.0220728634014,-80.2963964500695));
#30073=CARTESIAN_POINT('Ctrl Pts',(35.6813871324549,-30.0210841167044,-80.2896410310027));
#30074=CARTESIAN_POINT('Ctrl Pts',(35.6696916340288,-30.0201770928986,-80.2834439676601));
#30075=CARTESIAN_POINT('Ctrl Pts',(35.6580968184065,-30.019306721719,-80.277293533371));
#30076=CARTESIAN_POINT('Ctrl Pts',(35.6466609403558,-30.0184755468053,-80.2712210194501));
#30077=CARTESIAN_POINT('Ctrl Pts',(35.6358843219359,-30.0176922877635,-80.2654985760064));
#30078=CARTESIAN_POINT('Ctrl Pts',(35.6252491146204,-30.016943781666,-80.259845481224));
#30079=CARTESIAN_POINT('Ctrl Pts',(35.6147628037156,-30.0162286740995,-80.2542662512699));
#30080=CARTESIAN_POINT('Ctrl Pts',(35.6047424413365,-30.015545341608,-80.2489349287063));
#30081=CARTESIAN_POINT('Ctrl Pts',(35.5948582484425,-30.0148924602529,-80.2436711712074));
#30082=CARTESIAN_POINT('Ctrl Pts',(35.5850744769257,-30.0142662671988,-80.2384565839212));
#30083=CARTESIAN_POINT('Ctrl Pts',(35.5752147659519,-30.0136352137736,-80.2332015221691));
#30084=CARTESIAN_POINT('Ctrl Pts',(35.5654576226954,-30.0130312331291,-80.2279967106397));
#30085=CARTESIAN_POINT('Ctrl Pts',(35.5557161299514,-30.0124483251838,-80.2227966335814));
#30086=CARTESIAN_POINT('Ctrl Pts',(35.5463166337192,-30.011885881503,-80.2177791166565));
#30087=CARTESIAN_POINT('Ctrl Pts',(35.5369237555601,-30.0113425793404,-80.2127617960903));
#30088=CARTESIAN_POINT('Ctrl Pts',(35.527449210758,-30.0108138798861,-80.2076982897044));
#30089=CARTESIAN_POINT('Ctrl Pts',(35.5173854852471,-30.0102523029135,-80.2023199058924));
#30090=CARTESIAN_POINT('Ctrl Pts',(35.5072295820741,-30.0097072585674,-80.1968893857751));
#30091=CARTESIAN_POINT('Ctrl Pts',(35.4969314265015,-30.0091776938893,-80.1913806298767));
#30092=CARTESIAN_POINT('Ctrl Pts',(35.4863013363226,-30.0086310600534,-80.1856943133747));
#30093=CARTESIAN_POINT('Ctrl Pts',(35.4755200531343,-30.0081010145809,-80.179924829647));
#30094=CARTESIAN_POINT('Ctrl Pts',(35.4645869543455,-30.0075897005368,-80.1740723946893));
#30095=CARTESIAN_POINT('Ctrl Pts',(35.4529836026822,-30.0070470404201,-80.1678611766064));
#30096=CARTESIAN_POINT('Ctrl Pts',(35.4412095733346,-30.0065255874064,-80.1615566898743));
#30097=CARTESIAN_POINT('Ctrl Pts',(35.4293193553524,-30.006029968557,-80.155188639105));
#30098=CARTESIAN_POINT('Ctrl Pts',(35.4163900185768,-30.0054910362157,-80.1482640668957));
#30099=CARTESIAN_POINT('Ctrl Pts',(35.4033237830985,-30.0049828032927,-80.1412645884185));
#30100=CARTESIAN_POINT('Ctrl Pts',(35.390248088844,-30.0045114644718,-80.1342590949445));
#30101=CARTESIAN_POINT('Ctrl Pts',(35.3749727023187,-30.0039608334663,-80.1260750843265));
#30102=CARTESIAN_POINT('Ctrl Pts',(35.3596852987564,-30.0034608471724,-80.117883339593));
#30103=CARTESIAN_POINT('Ctrl Pts',(35.3446546541224,-30.0030178726731,-80.1098288811597));
#30104=CARTESIAN_POINT('Ctrl Pts',(35.3255177476667,-30.002453880791,-80.0995740037848));
#30105=CARTESIAN_POINT('Ctrl Pts',(35.3068025013319,-30.0019830567705,-80.0895446150785));
#30106=CARTESIAN_POINT('Ctrl Pts',(35.2891166492053,-30.0016033783673,-80.0800683623363));
#30107=CARTESIAN_POINT('Ctrl Pts',(35.2765328144717,-30.0013332296494,-80.0733258204701));
#30108=CARTESIAN_POINT('Ctrl Pts',(35.2644718949523,-30.001108780868,-80.0668642611809));
#30109=CARTESIAN_POINT('Ctrl Pts',(35.2531305794323,-30.0009240580503,-80.0607896234395));
#30110=CARTESIAN_POINT('Ctrl Pts',(35.2429440867967,-30.0007581445265,-80.055333532168));
#30111=CARTESIAN_POINT('Ctrl Pts',(35.2333387706015,-30.0006241571,-80.0501899303605));
#30112=CARTESIAN_POINT('Ctrl Pts',(35.2244232491389,-30.0005157480259,-80.0454172446047));
#30113=CARTESIAN_POINT('Ctrl Pts',(35.2160963048282,-30.0004144958079,-80.0409596378715));
#30114=CARTESIAN_POINT('Ctrl Pts',(35.2083714999213,-30.0003354840982,-80.0368258108517));
#30115=CARTESIAN_POINT('Ctrl Pts',(35.2012988663028,-30.0002729721797,-80.0330426119596));
#30116=CARTESIAN_POINT('Ctrl Pts',(35.194573831089,-30.0002135325317,-80.0294453457725));
#30117=CARTESIAN_POINT('Ctrl Pts',(35.1884387405858,-30.0001689686332,-80.026165250201));
#30118=CARTESIAN_POINT('Ctrl Pts',(35.1828955521313,-30.0001346028013,-80.0232032990606));
#30119=CARTESIAN_POINT('Ctrl Pts',(35.1772987906466,-30.0000999048353,-80.0202127216702));
#30120=CARTESIAN_POINT('Ctrl Pts',(35.1723061376744,-30.0000755729431,-80.0175468470756));
#30121=CARTESIAN_POINT('Ctrl Pts',(35.1678686123439,-30.0000576033295,-80.0151792621621));
#30122=CARTESIAN_POINT('Ctrl Pts',(35.1638451381212,-30.0000413104023,-80.0130325889241));
#30123=CARTESIAN_POINT('Ctrl Pts',(35.1602777470693,-30.0000302529948,-80.0111309837702));
#30124=CARTESIAN_POINT('Ctrl Pts',(35.1570869279604,-30.0000222392175,-80.0094316687598));
#30125=CARTESIAN_POINT('Ctrl Pts',(35.1539681240623,-30.0000144063073,-80.0077707064497));
#30126=CARTESIAN_POINT('Ctrl Pts',(35.1512092801205,-30.0000094851495,-80.0063031094198));
#30127=CARTESIAN_POINT('Ctrl Pts',(35.1486928450113,-30.0000061645488,-80.0049656980733));
#30128=CARTESIAN_POINT('Ctrl Pts',(35.1462489150872,-30.0000029396235,-80.0036668211031));
#30129=CARTESIAN_POINT('Ctrl Pts',(35.1440337268313,-30.0000012293401,-80.0024907891863));
#30130=CARTESIAN_POINT('Ctrl Pts',(35.1418962367331,-30.0000004600053,-80.0013564737718));
#30131=CARTESIAN_POINT('Ctrl Pts',(35.1410360151499,-30.0000001503906,-80.0008999745336));
#30132=CARTESIAN_POINT('Ctrl Pts',(35.1401878688062,-30.,-80.0004499589203));
#30133=CARTESIAN_POINT('Ctrl Pts',(35.1393398282202,-30.,-80.));
#30134=CARTESIAN_POINT('',(40.3554345327697,-32.0000000029374,-82.));
#30135=CARTESIAN_POINT('Ctrl Pts',(40.3554345313214,-32.0000000046471,-82.));
#30136=CARTESIAN_POINT('Ctrl Pts',(39.8311124520329,-31.5555126118589,-82.0000000010328));
#30137=CARTESIAN_POINT('Ctrl Pts',(38.4326846135015,-30.6269153251775,-81.6648999638687));
#30138=CARTESIAN_POINT('Ctrl Pts',(36.8259962365364,-30.1497856813059,-80.8876206939655));
#30139=CARTESIAN_POINT('Ctrl Pts',(35.9663031078275,-30.0488466897261,-80.4393185174872));
#30140=CARTESIAN_POINT('',(25.7,-32.,-82.));
#30141=CARTESIAN_POINT('Origin',(36.2,-30.,-82.));
#30142=CARTESIAN_POINT('',(-5.8,-30.,-60.5));
#30143=CARTESIAN_POINT('',(-5.8,-30.,-82.));
#30144=CARTESIAN_POINT('',(36.2,-30.,-60.5));
#30145=CARTESIAN_POINT('',(25.7,-30.,-60.5));
#30146=CARTESIAN_POINT('',(36.2,-30.,-79.4330532904862));
#30147=CARTESIAN_POINT('',(36.2,-30.,-82.));
#30148=CARTESIAN_POINT('',(35.6696699141101,-30.,-79.7165266452431));
#30149=CARTESIAN_POINT('Origin',(-5.79999999999999,-37.,-82.));
#30150=CARTESIAN_POINT('',(-12.8,-37.,-60.5));
#30151=CARTESIAN_POINT('',(-12.8,-37.,-82.));
#30152=CARTESIAN_POINT('Origin',(-5.79999999999999,-37.,-60.5));
#30153=CARTESIAN_POINT('Ctrl Pts',(43.1511535430799,-37.2336988749927,-80.4393174835207));
#30154=CARTESIAN_POINT('Ctrl Pts',(43.1518328407262,-37.239484438105,-80.4363004990864));
#30155=CARTESIAN_POINT('Ctrl Pts',(43.1531619914171,-37.251626360285,-80.4299516733943));
#30156=CARTESIAN_POINT('Ctrl Pts',(43.1616022519868,-37.3220234554072,-80.3933108331863));
#30157=CARTESIAN_POINT('Ctrl Pts',(43.1813231191454,-37.5335023841969,-80.2821011062626));
#30158=CARTESIAN_POINT('Ctrl Pts',(43.1946959334339,-37.760715809923,-80.1605544746364));
#30159=CARTESIAN_POINT('Ctrl Pts',(43.2000922890855,-37.9721391005235,-80.0472103209018));
#30160=CARTESIAN_POINT('Ctrl Pts',(43.1998885644922,-38.0426860747344,-80.0095380736286));
#30161=CARTESIAN_POINT('Ctrl Pts',(43.2,-38.0548562141931,-80.0030795017744));
#30162=CARTESIAN_POINT('Ctrl Pts',(43.2,-38.0606601717798,-80.));
#30163=CARTESIAN_POINT('Ctrl Pts',(43.1661027492299,-37.0769409045115,-80.1460536883894));
#30164=CARTESIAN_POINT('Ctrl Pts',(43.1664587837163,-37.0813561272506,-80.1437379532276));
#30165=CARTESIAN_POINT('Ctrl Pts',(43.1670812400941,-37.0893385332148,-80.1395507608468));
#30166=CARTESIAN_POINT('Ctrl Pts',(43.1731116841101,-37.1399593630532,-80.1133008325389));
#30167=CARTESIAN_POINT('Ctrl Pts',(43.1893842943803,-37.3106255658304,-80.0237140789211));
#30168=CARTESIAN_POINT('Ctrl Pts',(43.1981667671395,-37.4734287559457,-79.9363677700901));
#30169=CARTESIAN_POINT('Ctrl Pts',(43.2010845620737,-37.6439974687477,-79.8447395815119));
#30170=CARTESIAN_POINT('Ctrl Pts',(43.1999949346742,-37.6947024038551,-79.8176043851626));
#30171=CARTESIAN_POINT('Ctrl Pts',(43.2,-37.702687116552,-79.8133650160679));
#30172=CARTESIAN_POINT('Ctrl Pts',(43.2,-37.7071067811866,-79.8110177634954));
#30173=CARTESIAN_POINT('Ctrl Pts',(43.1810519553799,-36.9201829340303,-79.852789893258));
#30174=CARTESIAN_POINT('Ctrl Pts',(43.1811995800862,-36.9232120123378,-79.8511897097786));
#30175=CARTESIAN_POINT('Ctrl Pts',(43.1816990397624,-36.9308478545482,-79.8471474812294));
#30176=CARTESIAN_POINT('Ctrl Pts',(43.1844913922431,-36.9707931129032,-79.8259370685621));
#30177=CARTESIAN_POINT('Ctrl Pts',(43.1898784543209,-37.0722287967373,-79.7719437547884));
#30178=CARTESIAN_POINT('Ctrl Pts',(43.1966060738988,-37.2016426465078,-79.7030234840527));
#30179=CARTESIAN_POINT('Ctrl Pts',(43.1989499058728,-37.3029428680724,-79.6490065448319));
#30180=CARTESIAN_POINT('Ctrl Pts',(43.1998185084223,-37.3428746141862,-79.6277190373232));
#30181=CARTESIAN_POINT('Ctrl Pts',(43.2,-37.350518018911,-79.6236505303614));
#30182=CARTESIAN_POINT('Ctrl Pts',(43.2,-37.3535533905933,-79.6220355269908));
#30183=CARTESIAN_POINT('Ctrl Pts',(43.1960011615299,-36.7634249635491,-79.5595260981267));
#30184=CARTESIAN_POINT('Ctrl Pts',(43.196056955755,-36.7650749113605,-79.5586436598417));
#30185=CARTESIAN_POINT('Ctrl Pts',(43.1961660005796,-36.7685385217909,-79.5567913413279));
#30186=CARTESIAN_POINT('Ctrl Pts',(43.1968618855616,-36.7886560431392,-79.5460314243991));
#30187=CARTESIAN_POINT('Ctrl Pts',(43.1984815324142,-36.8491838061983,-79.5136657901732));
#30188=CARTESIAN_POINT('Ctrl Pts',(43.1995668915254,-36.9142231649016,-79.4789020799739));
#30189=CARTESIAN_POINT('Ctrl Pts',(43.2000074643706,-36.974740463544,-79.4465563376873));
#30190=CARTESIAN_POINT('Ctrl Pts',(43.1999908830157,-36.9948855968525,-79.4357877043179));
#30191=CARTESIAN_POINT('Ctrl Pts',(43.2,-36.99834892127,-79.4339360446549));
#30192=CARTESIAN_POINT('Ctrl Pts',(43.2,-37.,-79.4330532904862));
#30193=CARTESIAN_POINT('',(43.2,-38.0606601717798,-80.));
#30194=CARTESIAN_POINT('',(43.1511535430799,-37.2336988749927,-80.4393174835207));
#30195=CARTESIAN_POINT('Ctrl Pts',(43.2,-38.0606601717798,-80.));
#30196=CARTESIAN_POINT('Ctrl Pts',(43.2,-38.0585580345045,-80.0011153657436));
#30197=CARTESIAN_POINT('Ctrl Pts',(43.1999991196284,-38.0564519930821,-80.0022328244847));
#30198=CARTESIAN_POINT('Ctrl Pts',(43.1999970367979,-38.0541736842757,-80.003442789511));
#30199=CARTESIAN_POINT('Ctrl Pts',(43.1999949009836,-38.0518374190072,-80.0046835340753));
#30200=CARTESIAN_POINT('Ctrl Pts',(43.1999915030359,-38.0493201363092,-80.0060214842794));
#30201=CARTESIAN_POINT('Ctrl Pts',(43.1999858311707,-38.0464884913384,-80.0075282877598));
#30202=CARTESIAN_POINT('Ctrl Pts',(43.1999799943212,-38.0435744790187,-80.0090789213846));
#30203=CARTESIAN_POINT('Ctrl Pts',(43.1999717556759,-38.0403276954512,-80.0108082972709));
#30204=CARTESIAN_POINT('Ctrl Pts',(43.1999592405457,-38.0366511722259,-80.0127685612255));
#30205=CARTESIAN_POINT('Ctrl Pts',(43.1999460403082,-38.0327733875892,-80.0148361345771));
#30206=CARTESIAN_POINT('Ctrl Pts',(43.1999280866369,-38.0284175454673,-80.0171605574453));
#30207=CARTESIAN_POINT('Ctrl Pts',(43.1999022340605,-38.0235218920689,-80.0197750903894));
#30208=CARTESIAN_POINT('Ctrl Pts',(43.199875223834,-38.0184070166777,-80.0225066992529));
#30209=CARTESIAN_POINT('Ctrl Pts',(43.1998395772318,-38.0127031149793,-80.0255548701494));
#30210=CARTESIAN_POINT('Ctrl Pts',(43.1997907696175,-38.0063931646268,-80.0289288394644));
#30211=CARTESIAN_POINT('Ctrl Pts',(43.1997391599997,-37.9997209654207,-80.0324965054724));
#30212=CARTESIAN_POINT('Ctrl Pts',(43.1996727937424,-37.9923714094918,-80.0364283067011));
#30213=CARTESIAN_POINT('Ctrl Pts',(43.1995857188577,-37.9843791475729,-80.0407056868288));
#30214=CARTESIAN_POINT('Ctrl Pts',(43.1994916961757,-37.9757491746031,-80.0453243636512));
#30215=CARTESIAN_POINT('Ctrl Pts',(43.1993734426238,-37.966370232625,-80.0503457599974));
#30216=CARTESIAN_POINT('Ctrl Pts',(43.1992237896525,-37.9563431022343,-80.0557156969578));
#30217=CARTESIAN_POINT('Ctrl Pts',(43.1990546438421,-37.9450099019562,-80.0617850875693));
#30218=CARTESIAN_POINT('Ctrl Pts',(43.1988452035161,-37.9328493548553,-80.0682993586189));
#30219=CARTESIAN_POINT('Ctrl Pts',(43.198587751229,-37.9200694326044,-80.0751465277811));
#30220=CARTESIAN_POINT('Ctrl Pts',(43.1982019866816,-37.9009200943861,-80.085406273932));
#30221=CARTESIAN_POINT('Ctrl Pts',(43.1977069524981,-37.8803834507095,-80.0964116738306));
#30222=CARTESIAN_POINT('Ctrl Pts',(43.197096925486,-37.8592784408526,-80.1077212616636));
#30223=CARTESIAN_POINT('Ctrl Pts',(43.1966664800395,-37.8443863865487,-80.1157014994036));
#30224=CARTESIAN_POINT('Ctrl Pts',(43.1961794313092,-37.8292152691087,-80.123831066617));
#30225=CARTESIAN_POINT('Ctrl Pts',(43.1956415410083,-37.8140332294389,-80.1319652977188));
#30226=CARTESIAN_POINT('Ctrl Pts',(43.1951858481994,-37.8011712271138,-80.1388564995349));
#30227=CARTESIAN_POINT('Ctrl Pts',(43.1946938688436,-37.7883019867028,-80.1457507280178));
#30228=CARTESIAN_POINT('Ctrl Pts',(43.1941713808472,-37.7755522397004,-80.1525794999662));
#30229=CARTESIAN_POINT('Ctrl Pts',(43.1936920897984,-37.7638565841932,-80.1588436998935));
#30230=CARTESIAN_POINT('Ctrl Pts',(43.1931872432104,-37.752261854596,-80.1650526234636));
#30231=CARTESIAN_POINT('Ctrl Pts',(43.1926613511862,-37.7408263043073,-80.1711745877421));
#30232=CARTESIAN_POINT('Ctrl Pts',(43.1921657825137,-37.7300501369279,-80.1769435546995));
#30233=CARTESIAN_POINT('Ctrl Pts',(43.1916516129956,-37.7194155911391,-80.1826351629201));
#30234=CARTESIAN_POINT('Ctrl Pts',(43.1911212575987,-37.7089301959593,-80.1882448871515));
#30235=CARTESIAN_POINT('Ctrl Pts',(43.1906144722154,-37.6989107919042,-80.1936053044509));
#30236=CARTESIAN_POINT('Ctrl Pts',(43.1900929784067,-37.689027786831,-80.1988908477045));
#30237=CARTESIAN_POINT('Ctrl Pts',(43.1895564882148,-37.6792455207429,-80.2041200142135));
#30238=CARTESIAN_POINT('Ctrl Pts',(43.1890131220655,-37.6693378796787,-80.209416200636));
#30239=CARTESIAN_POINT('Ctrl Pts',(43.1884544776627,-37.6595342095919,-80.2146542275424));
#30240=CARTESIAN_POINT('Ctrl Pts',(43.1878764060617,-37.649746291343,-80.2198804089122));
#30241=CARTESIAN_POINT('Ctrl Pts',(43.1873214765315,-37.6403502150339,-80.224897369384));
#30242=CARTESIAN_POINT('Ctrl Pts',(43.1867481787444,-37.6309606427782,-80.2299076588121));
#30243=CARTESIAN_POINT('Ctrl Pts',(43.1861507982582,-37.6214895334211,-80.2349574569542));
#30244=CARTESIAN_POINT('Ctrl Pts',(43.1855161554004,-37.6114276515097,-80.2403222427113));
#30245=CARTESIAN_POINT('Ctrl Pts',(43.1848542702677,-37.6012737069304,-80.2457316334819));
#30246=CARTESIAN_POINT('Ctrl Pts',(43.1841604774403,-37.5909778004104,-80.2512114642367));
#30247=CARTESIAN_POINT('Ctrl Pts',(43.1834438932237,-37.5803436689861,-80.2568713097603));
#30248=CARTESIAN_POINT('Ctrl Pts',(43.1826932206741,-37.5695584681891,-80.2626060938773));
#30249=CARTESIAN_POINT('Ctrl Pts',(43.1819064399398,-37.5586217154527,-80.2684154677454));
#30250=CARTESIAN_POINT('Ctrl Pts',(43.181071384863,-37.5470139186443,-80.2745812861624));
#30251=CARTESIAN_POINT('Ctrl Pts',(43.1801955856503,-37.5352357254075,-80.280830944653));
#30252=CARTESIAN_POINT('Ctrl Pts',(43.1792810607772,-37.5233418532755,-80.287134955115));
#30253=CARTESIAN_POINT('Ctrl Pts',(43.1782865132751,-37.5104072451902,-80.2939905782281));
#30254=CARTESIAN_POINT('Ctrl Pts',(43.1772460744086,-37.4973363154097,-80.3009102024579));
#30255=CARTESIAN_POINT('Ctrl Pts',(43.1761688075758,-37.4842568799961,-80.3078259962454));
#30256=CARTESIAN_POINT('Ctrl Pts',(43.1749095786937,-37.4689681861163,-80.3159099425939));
#30257=CARTESIAN_POINT('Ctrl Pts',(43.1735998494352,-37.4536687660359,-80.3239881318433));
#30258=CARTESIAN_POINT('Ctrl Pts',(43.1722651888343,-37.4386284888155,-80.3319187022635));
#30259=CARTESIAN_POINT('Ctrl Pts',(43.1705695650427,-37.419520520939,-80.3419941205958));
#30260=CARTESIAN_POINT('Ctrl Pts',(43.1688336276888,-37.4008362912897,-80.3518282593479));
#30261=CARTESIAN_POINT('Ctrl Pts',(43.1671305083866,-37.3831816360191,-80.3611060273308));
#30262=CARTESIAN_POINT('Ctrl Pts',(43.1659173897706,-37.3706063625547,-80.3677145092148));
#30263=CARTESIAN_POINT('Ctrl Pts',(43.1647215545578,-37.3585552199351,-80.3740398813436));
#30264=CARTESIAN_POINT('Ctrl Pts',(43.1635718404781,-37.3472247949594,-80.3799810880577));
#30265=CARTESIAN_POINT('Ctrl Pts',(43.1625391128302,-37.337047270529,-80.3853177613607));
#30266=CARTESIAN_POINT('Ctrl Pts',(43.161543791978,-37.3274519135831,-80.3903441553375));
#30267=CARTESIAN_POINT('Ctrl Pts',(43.1606047204556,-37.3185472096877,-80.3950052279747));
#30268=CARTESIAN_POINT('Ctrl Pts',(43.1597276141756,-37.3102300884439,-80.3993587367162));
#30269=CARTESIAN_POINT('Ctrl Pts',(43.1588996965264,-37.3025158960185,-80.403393346525));
#30270=CARTESIAN_POINT('Ctrl Pts',(43.1581323377048,-37.2954544790796,-80.4070844482838));
#30271=CARTESIAN_POINT('Ctrl Pts',(43.1574026787078,-37.288739984821,-80.4105942086877));
#30272=CARTESIAN_POINT('Ctrl Pts',(43.1567278498295,-37.2826160035565,-80.4137932380386));
#30273=CARTESIAN_POINT('Ctrl Pts',(43.1561125509306,-37.2770842527928,-80.4166817587702));
#30274=CARTESIAN_POINT('Ctrl Pts',(43.1554921835504,-37.2715069346218,-80.4195940734879));
#30275=CARTESIAN_POINT('Ctrl Pts',(43.1549324406422,-37.2665323396178,-80.422190389511));
#30276=CARTESIAN_POINT('Ctrl Pts',(43.1544314048571,-37.2621113943169,-80.4244972128393));
#30277=CARTESIAN_POINT('Ctrl Pts',(43.153976437465,-37.2580969386355,-80.4265919322684));
#30278=CARTESIAN_POINT('Ctrl Pts',(43.1535698408209,-37.2545387286511,-80.4284480890782));
#30279=CARTESIAN_POINT('Ctrl Pts',(43.1532043757704,-37.2513569700072,-80.4301077382135));
#30280=CARTESIAN_POINT('Ctrl Pts',(43.1528471600527,-37.2482470305038,-80.4317299254958));
#30281=CARTESIAN_POINT('Ctrl Pts',(43.1525292589019,-37.2454969340214,-80.4331642750434));
#30282=CARTESIAN_POINT('Ctrl Pts',(43.1522381265435,-37.2429887872574,-80.4344724355697));
#30283=CARTESIAN_POINT('Ctrl Pts',(43.1519553742399,-37.2405528358604,-80.4357429415494));
#30284=CARTESIAN_POINT('Ctrl Pts',(43.1516978788855,-37.2383452067259,-80.4368943655259));
#30285=CARTESIAN_POINT('Ctrl Pts',(43.1514484584103,-37.2362144518533,-80.4380056097449));
#30286=CARTESIAN_POINT('Ctrl Pts',(43.1513493914683,-37.2353681405421,-80.4384469831588));
#30287=CARTESIAN_POINT('Ctrl Pts',(43.151251533532,-37.2345334575184,-80.4388822756696));
#30288=CARTESIAN_POINT('Ctrl Pts',(43.1511535430799,-37.2336988749927,-80.4393174835207));
#30289=CARTESIAN_POINT('',(43.1960011615299,-36.7634249635491,-79.5595260981267));
#30290=CARTESIAN_POINT('Ctrl Pts',(43.1960011615299,-36.7634249635491,-79.5595260981267));
#30291=CARTESIAN_POINT('Ctrl Pts',(43.1810519553799,-36.9201829340303,-79.852789893258));
#30292=CARTESIAN_POINT('Ctrl Pts',(43.1661027492299,-37.0769409045115,-80.1460536883894));
#30293=CARTESIAN_POINT('Ctrl Pts',(43.1511535430799,-37.2336988749927,-80.4393174835207));
#30294=CARTESIAN_POINT('',(43.2,-37.,-79.4330532904862));
#30295=CARTESIAN_POINT('Ctrl Pts',(43.1960011615299,-36.7634249635491,-79.5595260981267));
#30296=CARTESIAN_POINT('Ctrl Pts',(43.1960292081992,-36.7642543601491,-79.5590825136035));
#30297=CARTESIAN_POINT('Ctrl Pts',(43.1960572612725,-36.7650878480138,-79.5586367430988));
#30298=CARTESIAN_POINT('Ctrl Pts',(43.1960893558137,-36.7660475999897,-79.5581234426306));
#30299=CARTESIAN_POINT('Ctrl Pts',(43.1961226720754,-36.7670438861757,-79.5575906027109));
#30300=CARTESIAN_POINT('Ctrl Pts',(43.1961603389068,-36.7681760453388,-79.5569850937024));
#30301=CARTESIAN_POINT('Ctrl Pts',(43.1962049225249,-36.7695294334656,-79.5562612687486));
#30302=CARTESIAN_POINT('Ctrl Pts',(43.1962515944173,-36.7709462136155,-79.5555035401959));
#30303=CARTESIAN_POINT('Ctrl Pts',(43.1963058394868,-36.772605199104,-79.5546162773086));
#30304=CARTESIAN_POINT('Ctrl Pts',(43.1963685817354,-36.7745522931888,-79.5535749414745));
#30305=CARTESIAN_POINT('Ctrl Pts',(43.1964351400283,-36.7766178114237,-79.5524702705853));
#30306=CARTESIAN_POINT('Ctrl Pts',(43.1965112433384,-36.7790072392282,-79.5511923815391));
#30307=CARTESIAN_POINT('Ctrl Pts',(43.1965959455435,-36.781722253071,-79.5497403980796));
#30308=CARTESIAN_POINT('Ctrl Pts',(43.1966879807209,-36.7846723153569,-79.5481627112273));
#30309=CARTESIAN_POINT('Ctrl Pts',(43.196790129808,-36.7880063129438,-79.5463797305347));
#30310=CARTESIAN_POINT('Ctrl Pts',(43.1968992522861,-36.7916712853237,-79.5444198086112));
#30311=CARTESIAN_POINT('Ctrl Pts',(43.1970274016832,-36.7959752931622,-79.5421181488859));
#30312=CARTESIAN_POINT('Ctrl Pts',(43.1971650771572,-36.8007349526751,-79.5395728962987));
#30313=CARTESIAN_POINT('Ctrl Pts',(43.1973056544371,-36.8058001586425,-79.5368643638209));
#30314=CARTESIAN_POINT('Ctrl Pts',(43.1974945509819,-36.812606378731,-79.5332248537439));
#30315=CARTESIAN_POINT('Ctrl Pts',(43.1976882455755,-36.819958112586,-79.5292938352356));
#30316=CARTESIAN_POINT('Ctrl Pts',(43.1978725056392,-36.827430029207,-79.5252987932737));
#30317=CARTESIAN_POINT('Ctrl Pts',(43.1979954253998,-36.8324145396007,-79.5226337035527));
#30318=CARTESIAN_POINT('Ctrl Pts',(43.198114224774,-36.8374510429814,-79.5199409171317));
#30319=CARTESIAN_POINT('Ctrl Pts',(43.1982264691042,-36.8424364029054,-79.5172755779946));
#30320=CARTESIAN_POINT('Ctrl Pts',(43.1983273034174,-36.8469149840789,-79.5148811796236));
#30321=CARTESIAN_POINT('Ctrl Pts',(43.1984228681419,-36.8513517043665,-79.5125092451843));
#30322=CARTESIAN_POINT('Ctrl Pts',(43.1985126193353,-36.855704757511,-79.5101821187262));
#30323=CARTESIAN_POINT('Ctrl Pts',(43.1985964589664,-36.8597710919664,-79.5080082710417));
#30324=CARTESIAN_POINT('Ctrl Pts',(43.1986752428195,-36.8637640427497,-79.5058737234103));
#30325=CARTESIAN_POINT('Ctrl Pts',(43.1987493965147,-36.8676864149637,-79.5037769662875));
#30326=CARTESIAN_POINT('Ctrl Pts',(43.1988210097374,-36.8714744084558,-79.5017520431281));
#30327=CARTESIAN_POINT('Ctrl Pts',(43.1988883185089,-36.8751961754576,-79.4997625797108));
#30328=CARTESIAN_POINT('Ctrl Pts',(43.1989523298725,-36.8788955650162,-79.4977851230288));
#30329=CARTESIAN_POINT('Ctrl Pts',(43.199018439598,-36.8827162245807,-79.49574284317));
#30330=CARTESIAN_POINT('Ctrl Pts',(43.1990811576252,-36.8865194391444,-79.4937099356785));
#30331=CARTESIAN_POINT('Ctrl Pts',(43.1991415844903,-36.8903775558632,-79.4916477121475));
#30332=CARTESIAN_POINT('Ctrl Pts',(43.1992029440351,-36.8942952220383,-79.4895536585038));
#30333=CARTESIAN_POINT('Ctrl Pts',(43.1992619121571,-36.8982693617107,-79.4874294500976));
#30334=CARTESIAN_POINT('Ctrl Pts',(43.1993184857714,-36.9023233152792,-79.4852625997466));
#30335=CARTESIAN_POINT('Ctrl Pts',(43.1993790270456,-36.9066615835204,-79.4829437823496));
#30336=CARTESIAN_POINT('Ctrl Pts',(43.1994367895758,-36.9110908578823,-79.4805763437083));
#30337=CARTESIAN_POINT('Ctrl Pts',(43.1994909980028,-36.9155857306056,-79.4781738547406));
#30338=CARTESIAN_POINT('Ctrl Pts',(43.1995513398438,-36.9205891758262,-79.475499536093));
#30339=CARTESIAN_POINT('Ctrl Pts',(43.1996072226597,-36.9256732808927,-79.4727821198323));
#30340=CARTESIAN_POINT('Ctrl Pts',(43.1996574096079,-36.9307457718128,-79.4700709151224));
#30341=CARTESIAN_POINT('Ctrl Pts',(43.1997276363855,-36.937843726654,-79.4662771165926));
#30342=CARTESIAN_POINT('Ctrl Pts',(43.1997864800304,-36.9449173141003,-79.4624963497728));
#30343=CARTESIAN_POINT('Ctrl Pts',(43.1998327796822,-36.9516155346497,-79.4589161931795));
#30344=CARTESIAN_POINT('Ctrl Pts',(43.1998710512116,-36.9571523180866,-79.45595681739));
#30345=CARTESIAN_POINT('Ctrl Pts',(43.1999008268764,-36.962427686723,-79.4531371514988));
#30346=CARTESIAN_POINT('Ctrl Pts',(43.1999233926374,-36.9672509968511,-79.4505590813936));
#30347=CARTESIAN_POINT('Ctrl Pts',(43.1999421370943,-36.9712575237635,-79.4484175837531));
#30348=CARTESIAN_POINT('Ctrl Pts',(43.1999559634524,-36.9749512584795,-79.4464432532279));
#30349=CARTESIAN_POINT('Ctrl Pts',(43.1999662322813,-36.9782572558855,-79.4446761449678));
#30350=CARTESIAN_POINT('Ctrl Pts',(43.1999757221302,-36.9813124646361,-79.4430430872376));
#30351=CARTESIAN_POINT('Ctrl Pts',(43.1999821989834,-36.9840359420526,-79.441587320043));
#30352=CARTESIAN_POINT('Ctrl Pts',(43.1999868084131,-36.9864102228559,-79.4403181798015));
#30353=CARTESIAN_POINT('Ctrl Pts',(43.1999909974291,-36.9885679518936,-79.4391647944275));
#30354=CARTESIAN_POINT('Ctrl Pts',(43.1999936526081,-36.99043720414,-79.4381655845785));
#30355=CARTESIAN_POINT('Ctrl Pts',(43.1999954793619,-36.992044567104,-79.4373063422928));
#30356=CARTESIAN_POINT('Ctrl Pts',(43.1999972411365,-36.993594754739,-79.4364776640189));
#30357=CARTESIAN_POINT('Ctrl Pts',(43.1999982338138,-36.9949010490038,-79.4357793353878));
#30358=CARTESIAN_POINT('Ctrl Pts',(43.1999988737606,-36.9960291877518,-79.4351762236091));
#30359=CARTESIAN_POINT('Ctrl Pts',(43.1999994864524,-36.9971092795438,-79.4345987981081));
#30360=CARTESIAN_POINT('Ctrl Pts',(43.1999997736227,-36.9980259236369,-79.4341087287606));
#30361=CARTESIAN_POINT('Ctrl Pts',(43.1999999102358,-36.9988789739787,-79.4336526480419));
#30362=CARTESIAN_POINT('Ctrl Pts',(43.1999999713846,-36.9992608047016,-79.4334485034305));
#30363=CARTESIAN_POINT('Ctrl Pts',(43.2,-36.9996304850866,-79.433250852737));
#30364=CARTESIAN_POINT('Ctrl Pts',(43.2,-37.,-79.4330532904862));
#30365=CARTESIAN_POINT('',(43.2,-37.5303300858899,-79.7165266452431));
#30366=CARTESIAN_POINT('Ctrl Pts',(36.436577026206,-30.0039989057554,-79.5595271622931));
#30367=CARTESIAN_POINT('Ctrl Pts',(36.4332771028451,-30.0038873154276,-79.5577622708323));
#30368=CARTESIAN_POINT('Ctrl Pts',(36.4202666560633,-30.0033694511005,-79.5508025798716));
#30369=CARTESIAN_POINT('Ctrl Pts',(36.3506535373324,-30.0014962059641,-79.5135785874434));
#30370=CARTESIAN_POINT('Ctrl Pts',(36.2859379196174,-30.0004166770606,-79.4789881033753));
#30371=CARTESIAN_POINT('Ctrl Pts',(36.2163534620505,-29.9999221450745,-79.4417960806958));
#30372=CARTESIAN_POINT('Ctrl Pts',(36.2033021852651,-30.,-79.4348188136896));
#30373=CARTESIAN_POINT('Ctrl Pts',(36.2,-30.,-79.4330532904862));
#30374=CARTESIAN_POINT('Ctrl Pts',(36.2798190534131,-30.018948167079,-79.8527909473578));
#30375=CARTESIAN_POINT('Ctrl Pts',(36.2737608688324,-30.0186529125428,-79.8495905657678));
#30376=CARTESIAN_POINT('Ctrl Pts',(36.243977700825,-30.0168261623877,-79.8337978854855));
#30377=CARTESIAN_POINT('Ctrl Pts',(36.1277186009693,-30.0110875261413,-79.7718565459915));
#30378=CARTESIAN_POINT('Ctrl Pts',(35.9986160684372,-30.0048036635674,-79.7031095050481));
#30379=CARTESIAN_POINT('Ctrl Pts',(35.8823679293519,-30.0007586545453,-79.6411504032807));
#30380=CARTESIAN_POINT('Ctrl Pts',(35.8525173806862,-30.,-79.6252655486187));
#30381=CARTESIAN_POINT('Ctrl Pts',(35.8464466094067,-30.,-79.6220355269908));
#30382=CARTESIAN_POINT('Ctrl Pts',(36.1230610806203,-30.0338974284025,-80.1460547324225));
#30383=CARTESIAN_POINT('Ctrl Pts',(36.1142306075048,-30.0331853485277,-80.1414232481978));
#30384=CARTESIAN_POINT('Ctrl Pts',(36.0853799797672,-30.0285249362864,-80.1262758307435));
#30385=CARTESIAN_POINT('Ctrl Pts',(35.8888018779173,-30.0154387041423,-80.0204505126233));
#30386=CARTESIAN_POINT('Ctrl Pts',(35.7271314036452,-30.0041153121472,-79.9346805897903));
#30387=CARTESIAN_POINT('Ctrl Pts',(35.5307249156969,-30.0009916227304,-79.8304584379456));
#30388=CARTESIAN_POINT('Ctrl Pts',(35.5017325761074,-30.,-79.8157122835477));
#30389=CARTESIAN_POINT('Ctrl Pts',(35.4928932188134,-30.,-79.8110177634954));
#30390=CARTESIAN_POINT('Ctrl Pts',(35.9663031078275,-30.0488466897261,-80.4393185174872));
#30391=CARTESIAN_POINT('Ctrl Pts',(35.9547319536141,-30.0474880879196,-80.43328453461));
#30392=CARTESIAN_POINT('Ctrl Pts',(35.9091462718646,-30.0412136289532,-80.4097057710142));
#30393=CARTESIAN_POINT('Ctrl Pts',(35.6659250571246,-30.0184091986823,-80.2818326175006));
#30394=CARTESIAN_POINT('Ctrl Pts',(35.4398443483541,-30.0051041930071,-80.160865945828));
#30395=CARTESIAN_POINT('Ctrl Pts',(35.1967469144272,-29.9990469952302,-80.0305407044586));
#30396=CARTESIAN_POINT('Ctrl Pts',(35.1509477715285,-30.,-80.0061590184768));
#30397=CARTESIAN_POINT('Ctrl Pts',(35.1393398282202,-30.,-80.));
#30398=CARTESIAN_POINT('',(36.436577026206,-30.0039989057554,-79.5595271622931));
#30399=CARTESIAN_POINT('Ctrl Pts',(36.2,-30.,-79.4330532904862));
#30400=CARTESIAN_POINT('Ctrl Pts',(36.2008299527297,-30.,-79.4334970271891));
#30401=CARTESIAN_POINT('Ctrl Pts',(36.2016639947661,-30.0000001318966,-79.4339429495765));
#30402=CARTESIAN_POINT('Ctrl Pts',(36.2026243726041,-30.0000004919523,-79.4344563936253));
#30403=CARTESIAN_POINT('Ctrl Pts',(36.2036213072276,-30.0000008657134,-79.4349893819235));
#30404=CARTESIAN_POINT('Ctrl Pts',(36.2047541916982,-30.0000014834565,-79.4355950301953));
#30405=CARTESIAN_POINT('Ctrl Pts',(36.2061084253782,-30.0000026652048,-79.4363189798766));
#30406=CARTESIAN_POINT('Ctrl Pts',(36.2075260880269,-30.0000039023034,-79.4370768375772));
#30407=CARTESIAN_POINT('Ctrl Pts',(36.2091860867889,-30.0000057563249,-79.4379642132136));
#30408=CARTESIAN_POINT('Ctrl Pts',(36.2111343335543,-30.0000088552473,-79.4390056428516));
#30409=CARTESIAN_POINT('Ctrl Pts',(36.2132010681467,-30.0000121426389,-79.4401104098125));
#30410=CARTESIAN_POINT('Ctrl Pts',(36.2155918667794,-30.0000168376519,-79.4413883725556));
#30411=CARTESIAN_POINT('Ctrl Pts',(36.2183083747451,-30.0000239426542,-79.4428404082484));
#30412=CARTESIAN_POINT('Ctrl Pts',(36.2212600424038,-30.0000316627146,-79.4444181421803));
#30413=CARTESIAN_POINT('Ctrl Pts',(36.2245957852199,-30.0000422506377,-79.4462011421318));
#30414=CARTESIAN_POINT('Ctrl Pts',(36.2282625669554,-30.0000570554247,-79.4481610613737));
#30415=CARTESIAN_POINT('Ctrl Pts',(36.2325685639487,-30.0000744410705,-79.4504626454252));
#30416=CARTESIAN_POINT('Ctrl Pts',(36.2373302697605,-30.0000977058088,-79.4530077767654));
#30417=CARTESIAN_POINT('Ctrl Pts',(36.2423974506242,-30.0001283971647,-79.4557161645737));
#30418=CARTESIAN_POINT('Ctrl Pts',(36.2492077206762,-30.0001696462196,-79.4593562265481));
#30419=CARTESIAN_POINT('Ctrl Pts',(36.2565635895459,-30.0002245428704,-79.4632878753195));
#30420=CARTESIAN_POINT('Ctrl Pts',(36.2640392312156,-30.0002929363533,-79.4672835420005));
#30421=CARTESIAN_POINT('Ctrl Pts',(36.2690254529744,-30.0003385545207,-79.469948634982));
#30422=CARTESIAN_POINT('Ctrl Pts',(36.2740634720143,-30.0003900485922,-79.47264141353));
#30423=CARTESIAN_POINT('Ctrl Pts',(36.2790501104482,-30.0004463656574,-79.4753067399276));
#30424=CARTESIAN_POINT('Ctrl Pts',(36.2835298405669,-30.0004969579065,-79.4777011270678));
#30425=CARTESIAN_POINT('Ctrl Pts',(36.2879675194015,-30.0005514021085,-79.4800730463967));
#30426=CARTESIAN_POINT('Ctrl Pts',(36.2923213334954,-30.0006088285208,-79.4824001569821));
#30427=CARTESIAN_POINT('Ctrl Pts',(36.2963883789083,-30.0006624724802,-79.4845739899082));
#30428=CARTESIAN_POINT('Ctrl Pts',(36.3003818689944,-30.0007186889147,-79.4867085221443));
#30429=CARTESIAN_POINT('Ctrl Pts',(36.3043046120262,-30.0007771468605,-79.488805263923));
#30430=CARTESIAN_POINT('Ctrl Pts',(36.3080929712679,-30.0008336021769,-79.4908301763454));
#30431=CARTESIAN_POINT('Ctrl Pts',(36.31181494728,-30.0008921206218,-79.4928196289511));
#30432=CARTESIAN_POINT('Ctrl Pts',(36.3155143907173,-30.0009531773579,-79.4947970733165));
#30433=CARTESIAN_POINT('Ctrl Pts',(36.3193352828396,-30.0010162385198,-79.4968394350193));
#30434=CARTESIAN_POINT('Ctrl Pts',(36.3231385624469,-30.0010820990913,-79.4988724214067));
#30435=CARTESIAN_POINT('Ctrl Pts',(36.3269965827126,-30.0011521042404,-79.5009347253047));
#30436=CARTESIAN_POINT('Ctrl Pts',(36.3309140786862,-30.0012231885972,-79.5030288219293));
#30437=CARTESIAN_POINT('Ctrl Pts',(36.3348878788047,-30.0012985706632,-79.5051530737463));
#30438=CARTESIAN_POINT('Ctrl Pts',(36.338941318577,-30.001379042269,-79.5073199677846));
#30439=CARTESIAN_POINT('Ctrl Pts',(36.3432790352519,-30.0014651575305,-79.5096388310046));
#30440=CARTESIAN_POINT('Ctrl Pts',(36.3477075574441,-30.0015571244494,-79.5120063157128));
#30441=CARTESIAN_POINT('Ctrl Pts',(36.3522014777422,-30.0016548591704,-79.5144088482003));
#30442=CARTESIAN_POINT('Ctrl Pts',(36.3572038614396,-30.0017636520601,-79.5170832145777));
#30443=CARTESIAN_POINT('Ctrl Pts',(36.3622866553372,-30.0018796258686,-79.5198006753319));
#30444=CARTESIAN_POINT('Ctrl Pts',(36.3673576144516,-30.0020008981935,-79.5225119150777));
#30445=CARTESIAN_POINT('Ctrl Pts',(36.3744533378275,-30.0021705928904,-79.5263057155812));
#30446=CARTESIAN_POINT('Ctrl Pts',(36.3815242557079,-30.002350837276,-79.5300864658661));
#30447=CARTESIAN_POINT('Ctrl Pts',(36.3882195935254,-30.002530930071,-79.5336665752434));
#30448=CARTESIAN_POINT('Ctrl Pts',(36.3937541349189,-30.0026797994866,-79.5366259873123));
#30449=CARTESIAN_POINT('Ctrl Pts',(36.3990271081334,-30.0028283234338,-79.5394456612337));
#30450=CARTESIAN_POINT('Ctrl Pts',(36.403848040124,-30.0029687740773,-79.5420236987559));
#30451=CARTESIAN_POINT('Ctrl Pts',(36.4078525618013,-30.0030854398273,-79.5441651533881));
#30452=CARTESIAN_POINT('Ctrl Pts',(36.4115443102677,-30.003196448923,-79.5461394153452));
#30453=CARTESIAN_POINT('Ctrl Pts',(36.4148484404365,-30.0032979091831,-79.5479064272231));
#30454=CARTESIAN_POINT('Ctrl Pts',(36.4179018188432,-30.0033916695834,-79.5495393398617));
#30455=CARTESIAN_POINT('Ctrl Pts',(36.4206235917814,-30.003477230334,-79.5509949504925));
#30456=CARTESIAN_POINT('Ctrl Pts',(36.4229963509836,-30.0035528568103,-79.5522639251833));
#30457=CARTESIAN_POINT('Ctrl Pts',(36.4251527711832,-30.0036215879571,-79.553417199672));
#30458=CARTESIAN_POINT('Ctrl Pts',(36.4270208459444,-30.0036821028092,-79.5544162805173));
#30459=CARTESIAN_POINT('Ctrl Pts',(36.4286271741609,-30.0037345951404,-79.5552753797164));
#30460=CARTESIAN_POINT('Ctrl Pts',(36.4301763628356,-30.0037852202394,-79.5561039194482));
#30461=CARTESIAN_POINT('Ctrl Pts',(36.4314817914515,-30.0038283717003,-79.5568020965912));
#30462=CARTESIAN_POINT('Ctrl Pts',(36.4326091752435,-30.0038658552317,-79.5574050508185));
#30463=CARTESIAN_POINT('Ctrl Pts',(36.433688544672,-30.0039017423699,-79.5579823257132));
#30464=CARTESIAN_POINT('Ctrl Pts',(36.4346045677364,-30.0039324314054,-79.5584722388144));
#30465=CARTESIAN_POINT('Ctrl Pts',(36.4354570467087,-30.0039611222382,-79.5589281670262));
#30466=CARTESIAN_POINT('Ctrl Pts',(36.4358385180197,-30.0039739609473,-79.5591321879327));
#30467=CARTESIAN_POINT('Ctrl Pts',(36.4362078551915,-30.003986421855,-79.5593297192922));
#30468=CARTESIAN_POINT('Ctrl Pts',(36.4365770262059,-30.0039989057554,-79.5595271622931));
#30469=CARTESIAN_POINT('Ctrl Pts',(35.9663031078275,-30.0488466897261,-80.4393185174872));
#30470=CARTESIAN_POINT('Ctrl Pts',(36.1230610806203,-30.0338974284025,-80.1460547324225));
#30471=CARTESIAN_POINT('Ctrl Pts',(36.2798190534131,-30.018948167079,-79.8527909473578));
#30472=CARTESIAN_POINT('Ctrl Pts',(36.436577026206,-30.0039989057554,-79.5595271622931));
#30473=CARTESIAN_POINT('Ctrl Pts',(35.9663031078275,-30.0488466897261,-80.4393185174872));
#30474=CARTESIAN_POINT('Ctrl Pts',(36.8259962365364,-30.1497856813059,-80.8876206939655));
#30475=CARTESIAN_POINT('Ctrl Pts',(38.4326846135015,-30.6269153251775,-81.6648999638687));
#30476=CARTESIAN_POINT('Ctrl Pts',(39.8311124520329,-31.5555126118589,-82.0000000010328));
#30477=CARTESIAN_POINT('Ctrl Pts',(40.3554345313214,-32.0000000046471,-82.));
#30478=CARTESIAN_POINT('Ctrl Pts',(36.1230610806203,-30.0338974284025,-80.1460547324225));
#30479=CARTESIAN_POINT('Ctrl Pts',(36.9825844189037,-30.1108748191349,-80.598094697917));
#30480=CARTESIAN_POINT('Ctrl Pts',(38.5823256603806,-30.5454841504775,-81.4026214140165));
#30481=CARTESIAN_POINT('Ctrl Pts',(39.962810125821,-31.4492010715984,-81.7954256760992));
#30482=CARTESIAN_POINT('Ctrl Pts',(40.4786184794921,-31.8863889667545,-81.8224303038977));
#30483=CARTESIAN_POINT('Ctrl Pts',(36.2798190534131,-30.018948167079,-79.8527909473578));
#30484=CARTESIAN_POINT('Ctrl Pts',(37.139172601271,-30.0719639569638,-80.3085687018685));
#30485=CARTESIAN_POINT('Ctrl Pts',(38.7319667072597,-30.4640529757775,-81.1403428641643));
#30486=CARTESIAN_POINT('Ctrl Pts',(40.094507799609,-31.3428895313378,-81.5908513511656));
#30487=CARTESIAN_POINT('Ctrl Pts',(40.6018024276628,-31.7727779288618,-81.6448606077953));
#30488=CARTESIAN_POINT('Ctrl Pts',(36.436577026206,-30.0039989057554,-79.5595271622931));
#30489=CARTESIAN_POINT('Ctrl Pts',(37.2957607836383,-30.0330530947928,-80.01904270582));
#30490=CARTESIAN_POINT('Ctrl Pts',(38.8816077541387,-30.3826218010775,-80.8780643143121));
#30491=CARTESIAN_POINT('Ctrl Pts',(40.2262054733971,-31.2365779910773,-81.386277026232));
#30492=CARTESIAN_POINT('Ctrl Pts',(40.7249863758335,-31.6591668909691,-81.467290911693));
#30493=CARTESIAN_POINT('',(40.7249863758329,-31.6591668909686,-81.4672909116929));
#30494=CARTESIAN_POINT('Ctrl Pts',(36.436577026206,-30.0039989057554,-79.5595271622931));
#30495=CARTESIAN_POINT('Ctrl Pts',(37.2957607836383,-30.0330530947928,-80.01904270582));
#30496=CARTESIAN_POINT('Ctrl Pts',(38.8816077541387,-30.3826218010775,-80.8780643143121));
#30497=CARTESIAN_POINT('Ctrl Pts',(40.2262054733971,-31.2365779910773,-81.386277026232));
#30498=CARTESIAN_POINT('Ctrl Pts',(40.7249863758335,-31.6591668909691,-81.467290911693));
#30499=CARTESIAN_POINT('',(40.7249863758329,-31.6591668909686,-81.4672909116929));
#30500=CARTESIAN_POINT('Origin',(36.2,-37.,-81.75));
#30501=CARTESIAN_POINT('',(40.7490523794545,-32.3571428571429,-82.));
#30502=CARTESIAN_POINT('',(41.0989794855664,-32.,-81.5));
#30503=CARTESIAN_POINT('',(40.7490523794545,-32.3571428571429,-82.));
#30504=CARTESIAN_POINT('',(41.2,-32.1010205144336,-81.5));
#30505=CARTESIAN_POINT('Origin',(36.2,-37.,-81.5));
#30506=CARTESIAN_POINT('',(40.8428571428571,-32.4509476205455,-82.));
#30507=CARTESIAN_POINT('',(41.2,-32.1010205144336,-81.5));
#30508=CARTESIAN_POINT('Origin',(36.2,-37.,-82.));
#30509=CARTESIAN_POINT('Ctrl Pts',(40.3554345313208,-32.0000000046466,-82.));
#30510=CARTESIAN_POINT('Ctrl Pts',(40.4919662599274,-32.1157430459277,-82.));
#30511=CARTESIAN_POINT('Ctrl Pts',(40.6227896098978,-32.2334311135731,-82.));
#30512=CARTESIAN_POINT('Ctrl Pts',(40.7490523794545,-32.3571428571429,-82.));
#30513=CARTESIAN_POINT('Ctrl Pts',(40.4786184794915,-31.8863889667539,-81.8224303038976));
#30514=CARTESIAN_POINT('Ctrl Pts',(40.6129332622184,-32.0002312430992,-81.8294622194963));
#30515=CARTESIAN_POINT('Ctrl Pts',(40.7417444835387,-32.1166492773747,-81.8333333333333));
#30516=CARTESIAN_POINT('Ctrl Pts',(40.8656947481584,-32.2380952380952,-81.8333333333333));
#30517=CARTESIAN_POINT('Ctrl Pts',(40.6018024276622,-31.7727779288612,-81.6448606077953));
#30518=CARTESIAN_POINT('Ctrl Pts',(40.7339002645095,-31.8847194402708,-81.6589244389925));
#30519=CARTESIAN_POINT('Ctrl Pts',(40.8606993571796,-31.9998674411764,-81.6666666666667));
#30520=CARTESIAN_POINT('Ctrl Pts',(40.9823371168624,-32.1190476190476,-81.6666666666667));
#30521=CARTESIAN_POINT('Ctrl Pts',(40.7249863758329,-31.6591668909686,-81.4672909116929));
#30522=CARTESIAN_POINT('Ctrl Pts',(40.8548672668006,-31.7692076374424,-81.4883866584888));
#30523=CARTESIAN_POINT('Ctrl Pts',(40.9796542308205,-31.883085604978,-81.5));
#30524=CARTESIAN_POINT('Ctrl Pts',(41.0989794855664,-32.,-81.5));
#30525=CARTESIAN_POINT('Ctrl Pts',(40.7490523794545,-32.3571428571429,-82.));
#30526=CARTESIAN_POINT('Ctrl Pts',(40.6227896098978,-32.2334311135731,-82.));
#30527=CARTESIAN_POINT('Ctrl Pts',(40.4919662599274,-32.1157430459277,-82.));
#30528=CARTESIAN_POINT('Ctrl Pts',(40.3554345313208,-32.0000000046466,-82.));
#30529=CARTESIAN_POINT('Ctrl Pts',(40.7249863758329,-31.6591668909686,-81.4672909116929));
#30530=CARTESIAN_POINT('Ctrl Pts',(40.8548672668006,-31.7692076374424,-81.4883866584888));
#30531=CARTESIAN_POINT('Ctrl Pts',(40.9796542308205,-31.883085604978,-81.5));
#30532=CARTESIAN_POINT('Ctrl Pts',(41.0989794855664,-32.,-81.5));
#30533=CARTESIAN_POINT('Ctrl Pts',(41.1999999953529,-32.8445654686786,-82.));
#30534=CARTESIAN_POINT('Ctrl Pts',(41.6444875838123,-33.3688877787829,-82.0000000010328));
#30535=CARTESIAN_POINT('Ctrl Pts',(42.5730840238607,-34.7673153509566,-81.6649014644068));
#30536=CARTESIAN_POINT('Ctrl Pts',(43.0502156814288,-36.3740133275242,-80.8876157502161));
#30537=CARTESIAN_POINT('Ctrl Pts',(43.1511535430799,-37.2336988749927,-80.4393174835207));
#30538=CARTESIAN_POINT('Ctrl Pts',(41.3136110332456,-32.7213815205079,-81.8224303038976));
#30539=CARTESIAN_POINT('Ctrl Pts',(41.7507991208595,-33.237190101247,-81.7954256642113));
#30540=CARTESIAN_POINT('Ctrl Pts',(42.6545151103675,-34.6176754805104,-81.4026223559956));
#30541=CARTESIAN_POINT('Ctrl Pts',(43.0891261012142,-36.217419896311,-80.5980924994436));
#30542=CARTESIAN_POINT('Ctrl Pts',(43.1661027492299,-37.0769409045115,-80.1460536883894));
#30543=CARTESIAN_POINT('Ctrl Pts',(41.4272220711382,-32.5981975723372,-81.6448606077953));
#30544=CARTESIAN_POINT('Ctrl Pts',(41.8571106579067,-33.1054924237111,-81.5908513273897));
#30545=CARTESIAN_POINT('Ctrl Pts',(42.7359461968743,-34.4680356100643,-81.1403432475844));
#30546=CARTESIAN_POINT('Ctrl Pts',(43.1280365209996,-36.0608264650977,-80.308569248671));
#30547=CARTESIAN_POINT('Ctrl Pts',(43.1810519553799,-36.9201829340303,-79.852789893258));
#30548=CARTESIAN_POINT('Ctrl Pts',(41.5408331090309,-32.4750136241665,-81.467290911693));
#30549=CARTESIAN_POINT('Ctrl Pts',(41.9634221949539,-32.9737947461752,-81.3862769905682));
#30550=CARTESIAN_POINT('Ctrl Pts',(42.8173772833811,-34.3183957396181,-80.8780641391733));
#30551=CARTESIAN_POINT('Ctrl Pts',(43.166946940785,-35.9042330338845,-80.0190459978984));
#30552=CARTESIAN_POINT('Ctrl Pts',(43.1960011615299,-36.7634249635491,-79.5595260981267));
#30553=CARTESIAN_POINT('',(41.1999999970626,-32.8445654672303,-82.));
#30554=CARTESIAN_POINT('Ctrl Pts',(43.1511535430799,-37.2336988749927,-80.4393174835207));
#30555=CARTESIAN_POINT('Ctrl Pts',(43.0502156814288,-36.3740133275242,-80.8876157502161));
#30556=CARTESIAN_POINT('Ctrl Pts',(42.5730840238607,-34.7673153509566,-81.6649014644068));
#30557=CARTESIAN_POINT('Ctrl Pts',(41.6444875838123,-33.3688877787829,-82.0000000010328));
#30558=CARTESIAN_POINT('Ctrl Pts',(41.1999999953529,-32.8445654686786,-82.));
#30559=CARTESIAN_POINT('',(41.5408331090314,-32.4750136241671,-81.4672909116929));
#30560=CARTESIAN_POINT('',(41.1999999970626,-32.8445654672303,-82.));
#30561=CARTESIAN_POINT('Ctrl Pts',(41.5408331090309,-32.4750136241665,-81.467290911693));
#30562=CARTESIAN_POINT('Ctrl Pts',(41.9634221949539,-32.9737947461752,-81.3862769905682));
#30563=CARTESIAN_POINT('Ctrl Pts',(42.8173772833811,-34.3183957396181,-80.8780641391733));
#30564=CARTESIAN_POINT('Ctrl Pts',(43.166946940785,-35.9042330338845,-80.0190459978984));
#30565=CARTESIAN_POINT('Ctrl Pts',(43.1960011615299,-36.7634249635491,-79.5595260981267));
#30566=CARTESIAN_POINT('Ctrl Pts',(40.8428571428571,-32.4509476205455,-82.));
#30567=CARTESIAN_POINT('Ctrl Pts',(40.9665688864269,-32.5772103901022,-82.));
#30568=CARTESIAN_POINT('Ctrl Pts',(41.0842569540723,-32.7080337400726,-82.));
#30569=CARTESIAN_POINT('Ctrl Pts',(41.1999999953534,-32.8445654686792,-82.));
#30570=CARTESIAN_POINT('Ctrl Pts',(40.9619047619048,-32.3343052518416,-81.8333333333333));
#30571=CARTESIAN_POINT('Ctrl Pts',(41.0833507226253,-32.4582555164613,-81.8333333333333));
#30572=CARTESIAN_POINT('Ctrl Pts',(41.1997687569007,-32.5870667377815,-81.8294622194963));
#30573=CARTESIAN_POINT('Ctrl Pts',(41.3136110332461,-32.7213815205085,-81.8224303038976));
#30574=CARTESIAN_POINT('Ctrl Pts',(41.0809523809524,-32.2176628831376,-81.6666666666667));
#30575=CARTESIAN_POINT('Ctrl Pts',(41.2001325588236,-32.3393006428204,-81.6666666666667));
#30576=CARTESIAN_POINT('Ctrl Pts',(41.3152805597292,-32.4660997354905,-81.6589244389925));
#30577=CARTESIAN_POINT('Ctrl Pts',(41.4272220711388,-32.5981975723378,-81.6448606077953));
#30578=CARTESIAN_POINT('Ctrl Pts',(41.2,-32.1010205144336,-81.5));
#30579=CARTESIAN_POINT('Ctrl Pts',(41.316914395022,-32.2203457691795,-81.5));
#30580=CARTESIAN_POINT('Ctrl Pts',(41.4307923625576,-32.3451327331994,-81.4883866584888));
#30581=CARTESIAN_POINT('Ctrl Pts',(41.5408331090314,-32.4750136241671,-81.4672909116929));
#30582=CARTESIAN_POINT('Ctrl Pts',(41.1999999953534,-32.8445654686792,-82.));
#30583=CARTESIAN_POINT('Ctrl Pts',(41.0842569540723,-32.7080337400726,-82.));
#30584=CARTESIAN_POINT('Ctrl Pts',(40.9665688864269,-32.5772103901022,-82.));
#30585=CARTESIAN_POINT('Ctrl Pts',(40.8428571428571,-32.4509476205455,-82.));
#30586=CARTESIAN_POINT('Ctrl Pts',(41.2,-32.1010205144336,-81.5));
#30587=CARTESIAN_POINT('Ctrl Pts',(41.316914395022,-32.2203457691795,-81.5));
#30588=CARTESIAN_POINT('Ctrl Pts',(41.4307923625576,-32.3451327331994,-81.4883866584888));
#30589=CARTESIAN_POINT('Ctrl Pts',(41.5408331090314,-32.4750136241671,-81.4672909116929));
#30590=CARTESIAN_POINT('Origin',(15.2,-53.,-82.));
#30591=CARTESIAN_POINT('',(41.1999999970626,-73.1554345327697,-82.));
#30592=CARTESIAN_POINT('',(41.2,-61.,-82.));
#30593=CARTESIAN_POINT('',(40.8428571428571,-73.5490523794545,-82.));
#30594=CARTESIAN_POINT('Ctrl Pts',(40.8428571428571,-73.5490523794545,-82.));
#30595=CARTESIAN_POINT('Ctrl Pts',(40.9665688864269,-73.4227896098978,-82.));
#30596=CARTESIAN_POINT('Ctrl Pts',(41.0842569540723,-73.2919662599274,-82.));
#30597=CARTESIAN_POINT('Ctrl Pts',(41.1999999953534,-73.1554345313208,-82.));
#30598=CARTESIAN_POINT('',(40.7490523794545,-73.6428571428571,-82.));
#30599=CARTESIAN_POINT('Origin',(36.2,-69.,-82.));
#30600=CARTESIAN_POINT('',(40.3554345327697,-73.9999999970625,-82.));
#30601=CARTESIAN_POINT('Ctrl Pts',(40.3554345313208,-73.9999999953534,-82.));
#30602=CARTESIAN_POINT('Ctrl Pts',(40.4919662599274,-73.8842569540723,-82.));
#30603=CARTESIAN_POINT('Ctrl Pts',(40.6227896098978,-73.7665688864269,-82.));
#30604=CARTESIAN_POINT('Ctrl Pts',(40.7490523794545,-73.6428571428571,-82.));
#30605=CARTESIAN_POINT('',(-9.95543453276968,-73.9999999970625,-82.));
#30606=CARTESIAN_POINT('',(4.7,-74.,-82.));
#30607=CARTESIAN_POINT('',(-10.3490523794545,-73.6428571428571,-82.));
#30608=CARTESIAN_POINT('Ctrl Pts',(-10.3490523794545,-73.6428571428571,
-82.));
#30609=CARTESIAN_POINT('Ctrl Pts',(-10.2227896098978,-73.7665688864269,
-82.));
#30610=CARTESIAN_POINT('Ctrl Pts',(-10.0919662599274,-73.8842569540723,
-82.));
#30611=CARTESIAN_POINT('Ctrl Pts',(-9.95543453132077,-73.9999999953534,
-82.));
#30612=CARTESIAN_POINT('',(-10.4428571428571,-73.5490523794545,-82.));
#30613=CARTESIAN_POINT('Origin',(-5.8,-69.,-82.));
#30614=CARTESIAN_POINT('',(-10.7999999970626,-73.1554345327697,-82.));
#30615=CARTESIAN_POINT('Ctrl Pts',(-10.7999999953534,-73.1554345313208,
-82.));
#30616=CARTESIAN_POINT('Ctrl Pts',(-10.6842569540723,-73.2919662599274,
-82.));
#30617=CARTESIAN_POINT('Ctrl Pts',(-10.5665688864269,-73.4227896098978,
-82.));
#30618=CARTESIAN_POINT('Ctrl Pts',(-10.4428571428571,-73.5490523794545,
-82.));
#30619=CARTESIAN_POINT('',(-10.8,-45.,-82.));
#30620=CARTESIAN_POINT('Origin',(6.2,-75.5,-12.5));
#30621=CARTESIAN_POINT('',(6.7,-76.,-12.5));
#30622=CARTESIAN_POINT('',(6.7,-75.5,-12.));
#30623=CARTESIAN_POINT('',(6.7,-76.,-12.5));
#30624=CARTESIAN_POINT('Origin',(9.2,-75.75,-12.25));
#30625=CARTESIAN_POINT('',(23.7,-76.,-12.5));
#30626=CARTESIAN_POINT('',(9.2,-76.,-12.5));
#30627=CARTESIAN_POINT('',(23.7,-76.,-12.5));
#30628=CARTESIAN_POINT('Origin',(4.7,-75.75,-60.25));
#30629=CARTESIAN_POINT('',(23.7,-76.,-60.5));
#30630=CARTESIAN_POINT('',(36.2,-76.,-60.5));
#30631=CARTESIAN_POINT('',(4.7,-76.,-60.5));
#30632=CARTESIAN_POINT('',(36.2,-76.,-60.5));
#30633=CARTESIAN_POINT('',(24.2,-75.5,-60.));
#30634=CARTESIAN_POINT('Origin',(36.2,-69.,-60.25));
#30635=CARTESIAN_POINT('',(43.2,-69.,-60.5));
#30636=CARTESIAN_POINT('',(43.2,-69.,-60.5));
#30637=CARTESIAN_POINT('Origin',(36.2,-69.,-60.5));
#30638=CARTESIAN_POINT('Origin',(42.95,-61.,-60.25));
#30639=CARTESIAN_POINT('',(43.2,-37.,-60.5));
#30640=CARTESIAN_POINT('',(43.2,-37.,-60.5));
#30641=CARTESIAN_POINT('',(43.2,-61.,-60.5));
#30642=CARTESIAN_POINT('Origin',(36.2,-37.,-60.25));
#30643=CARTESIAN_POINT('',(36.2,-30.,-60.5));
#30644=CARTESIAN_POINT('Origin',(36.2,-37.,-60.5));
#30645=CARTESIAN_POINT('Origin',(25.7,-30.25,-60.25));
#30646=CARTESIAN_POINT('',(-5.8,-30.,-60.5));
#30647=CARTESIAN_POINT('Origin',(-5.79999999999999,-37.,-60.25));
#30648=CARTESIAN_POINT('',(-12.8,-37.,-60.5));
#30649=CARTESIAN_POINT('Origin',(-12.55,-45.,-60.25));
#30650=CARTESIAN_POINT('',(-12.8,-69.,-60.5));
#30651=CARTESIAN_POINT('',(-12.8,-69.,-60.5));
#30652=CARTESIAN_POINT('',(-12.8,-45.,-60.5));
#30653=CARTESIAN_POINT('Origin',(-5.8,-69.,-60.25));
#30654=CARTESIAN_POINT('',(-5.8,-76.,-60.5));
#30655=CARTESIAN_POINT('',(-5.8,-76.,-60.5));
#30656=CARTESIAN_POINT('Origin',(-5.8,-69.,-60.5));
#30657=CARTESIAN_POINT('Origin',(4.7,-75.75,-60.25));
#30658=CARTESIAN_POINT('',(6.7,-76.,-60.5));
#30659=CARTESIAN_POINT('',(4.7,-76.,-60.5));
#30660=CARTESIAN_POINT('',(6.7,-76.,-60.5));
#30661=CARTESIAN_POINT('Origin',(23.95,-75.75,-74.));
#30662=CARTESIAN_POINT('',(23.7,-76.,-74.));
#30663=CARTESIAN_POINT('',(24.2,-75.5,-74.));
#30664=CARTESIAN_POINT('Origin',(6.45,-75.75,-47.));
#30665=CARTESIAN_POINT('',(6.7,-76.,-47.));
#30666=CARTESIAN_POINT('',(6.2,-75.5,-47.));
#30667=CARTESIAN_POINT('Origin',(36.2,-37.,-82.));
#30668=CARTESIAN_POINT('',(43.2,-37.,-82.));
#30669=CARTESIAN_POINT('Origin',(43.2,-69.,-82.));
#30670=CARTESIAN_POINT('',(43.2,-69.,-79.4330532904862));
#30671=CARTESIAN_POINT('',(43.2,-69.,-82.));
#30672=CARTESIAN_POINT('',(43.2,-67.9393398282202,-80.));
#30673=CARTESIAN_POINT('',(43.2,-68.4696699141101,-79.7165266452431));
#30674=CARTESIAN_POINT('',(43.2,-61.,-80.));
#30675=CARTESIAN_POINT('Origin',(36.2,-69.,-82.));
#30676=CARTESIAN_POINT('',(36.2,-76.,-79.4330532904862));
#30677=CARTESIAN_POINT('',(36.2,-76.,-82.));
#30678=CARTESIAN_POINT('',(36.436575036449,-75.99600116153,-79.5595260981257));
#30679=CARTESIAN_POINT('Ctrl Pts',(36.436575036449,-75.99600116153,-79.5595260981258));
#30680=CARTESIAN_POINT('Ctrl Pts',(36.4357456398491,-75.9960292081993,-79.5590825136025));
#30681=CARTESIAN_POINT('Ctrl Pts',(36.4349121519844,-75.9960572612725,-79.5586367430978));
#30682=CARTESIAN_POINT('Ctrl Pts',(36.4339524000084,-75.9960893558137,-79.5581234426296));
#30683=CARTESIAN_POINT('Ctrl Pts',(36.4329561138224,-75.9961226720755,-79.55759060271));
#30684=CARTESIAN_POINT('Ctrl Pts',(36.4318239546593,-75.9961603389068,-79.5569850937014));
#30685=CARTESIAN_POINT('Ctrl Pts',(36.4304705665326,-75.9962049225249,-79.5562612687477));
#30686=CARTESIAN_POINT('Ctrl Pts',(36.4290537863826,-75.9962515944174,-79.555503540195));
#30687=CARTESIAN_POINT('Ctrl Pts',(36.4273948008941,-75.9963058394869,-79.5546162773077));
#30688=CARTESIAN_POINT('Ctrl Pts',(36.4254477068093,-75.9963685817354,-79.5535749414736));
#30689=CARTESIAN_POINT('Ctrl Pts',(36.4233821885744,-75.9964351400283,-79.5524702705845));
#30690=CARTESIAN_POINT('Ctrl Pts',(36.4209927607699,-75.9965112433385,-79.5511923815383));
#30691=CARTESIAN_POINT('Ctrl Pts',(36.4182777469271,-75.9965959455435,-79.5497403980789));
#30692=CARTESIAN_POINT('Ctrl Pts',(36.4153276846412,-75.9966879807209,-79.5481627112266));
#30693=CARTESIAN_POINT('Ctrl Pts',(36.4119936870543,-75.996790129808,-79.5463797305341));
#30694=CARTESIAN_POINT('Ctrl Pts',(36.4083287146744,-75.9968992522861,-79.5444198086106));
#30695=CARTESIAN_POINT('Ctrl Pts',(36.4040247068359,-75.9970274016833,-79.5421181488853));
#30696=CARTESIAN_POINT('Ctrl Pts',(36.3992650473229,-75.9971650771572,-79.5395728962982));
#30697=CARTESIAN_POINT('Ctrl Pts',(36.3941998413555,-75.9973056544371,-79.5368643638204));
#30698=CARTESIAN_POINT('Ctrl Pts',(36.3873936212671,-75.997494550982,-79.5332248537436));
#30699=CARTESIAN_POINT('Ctrl Pts',(36.3800418874122,-75.9976882455756,-79.5292938352354));
#30700=CARTESIAN_POINT('Ctrl Pts',(36.3725699707913,-75.9978725056392,-79.5252987932736));
#30701=CARTESIAN_POINT('Ctrl Pts',(36.3675854603976,-75.9979954253998,-79.5226337035528));
#30702=CARTESIAN_POINT('Ctrl Pts',(36.3625489570169,-75.9981142247741,-79.5199409171318));
#30703=CARTESIAN_POINT('Ctrl Pts',(36.3575635970929,-75.9982264691042,-79.5172755779947));
#30704=CARTESIAN_POINT('Ctrl Pts',(36.3530850159194,-75.9983273034174,-79.5148811796238));
#30705=CARTESIAN_POINT('Ctrl Pts',(36.3486482956318,-75.998422868142,-79.5125092451845));
#30706=CARTESIAN_POINT('Ctrl Pts',(36.3442952424874,-75.9985126193353,-79.5101821187264));
#30707=CARTESIAN_POINT('Ctrl Pts',(36.340228908032,-75.9985964589664,-79.508008271042));
#30708=CARTESIAN_POINT('Ctrl Pts',(36.3362359572487,-75.9986752428195,-79.5058737234106));
#30709=CARTESIAN_POINT('Ctrl Pts',(36.3323135850348,-75.9987493965147,-79.5037769662878));
#30710=CARTESIAN_POINT('Ctrl Pts',(36.3285255915427,-75.9988210097374,-79.5017520431284));
#30711=CARTESIAN_POINT('Ctrl Pts',(36.324803824541,-75.9988883185089,-79.4997625797111));
#30712=CARTESIAN_POINT('Ctrl Pts',(36.3211044349824,-75.9989523298725,-79.4977851230291));
#30713=CARTESIAN_POINT('Ctrl Pts',(36.3172837754179,-75.9990184395981,-79.4957428431703));
#30714=CARTESIAN_POINT('Ctrl Pts',(36.3134805608543,-75.9990811576252,-79.4937099356788));
#30715=CARTESIAN_POINT('Ctrl Pts',(36.3096224441355,-75.9991415844903,-79.4916477121478));
#30716=CARTESIAN_POINT('Ctrl Pts',(36.3057047779605,-75.9992029440351,-79.4895536585041));
#30717=CARTESIAN_POINT('Ctrl Pts',(36.301730638288,-75.9992619121571,-79.4874294500978));
#30718=CARTESIAN_POINT('Ctrl Pts',(36.2976766847196,-75.9993184857715,-79.4852625997468));
#30719=CARTESIAN_POINT('Ctrl Pts',(36.2933384164784,-75.9993790270456,-79.4829437823498));
#30720=CARTESIAN_POINT('Ctrl Pts',(36.2889091421166,-75.9994367895758,-79.4805763437085));
#30721=CARTESIAN_POINT('Ctrl Pts',(36.2844142693933,-75.9994909980028,-79.4781738547408));
#30722=CARTESIAN_POINT('Ctrl Pts',(36.2794108241728,-75.9995513398438,-79.4754995360931));
#30723=CARTESIAN_POINT('Ctrl Pts',(36.2743267191064,-75.9996072226597,-79.4727821198323));
#30724=CARTESIAN_POINT('Ctrl Pts',(36.2692542281862,-75.9996574096079,-79.4700709151225));
#30725=CARTESIAN_POINT('Ctrl Pts',(36.262156273345,-75.9997276363855,-79.4662771165925));
#30726=CARTESIAN_POINT('Ctrl Pts',(36.2550826858987,-75.9997864800304,-79.4624963497726));
#30727=CARTESIAN_POINT('Ctrl Pts',(36.2483844653493,-75.9998327796822,-79.4589161931793));
#30728=CARTESIAN_POINT('Ctrl Pts',(36.2428476819125,-75.9998710512116,-79.4559568173898));
#30729=CARTESIAN_POINT('Ctrl Pts',(36.2375723132762,-75.9999008268764,-79.4531371514986));
#30730=CARTESIAN_POINT('Ctrl Pts',(36.2327490031482,-75.9999233926374,-79.4505590813934));
#30731=CARTESIAN_POINT('Ctrl Pts',(36.2287424762358,-75.9999421370944,-79.4484175837529));
#30732=CARTESIAN_POINT('Ctrl Pts',(36.2250487415199,-75.9999559634524,-79.4464432532277));
#30733=CARTESIAN_POINT('Ctrl Pts',(36.221742744114,-75.9999662322813,-79.4446761449676));
#30734=CARTESIAN_POINT('Ctrl Pts',(36.2186875353634,-75.9999757221302,-79.4430430872375));
#30735=CARTESIAN_POINT('Ctrl Pts',(36.2159640579471,-75.9999821989834,-79.4415873200428));
#30736=CARTESIAN_POINT('Ctrl Pts',(36.2135897771439,-75.9999868084131,-79.4403181798014));
#30737=CARTESIAN_POINT('Ctrl Pts',(36.2114320481061,-75.9999909974291,-79.4391647944274));
#30738=CARTESIAN_POINT('Ctrl Pts',(36.2095627958598,-75.9999936526082,-79.4381655845784));
#30739=CARTESIAN_POINT('Ctrl Pts',(36.2079554328958,-75.9999954793619,-79.4373063422927));
#30740=CARTESIAN_POINT('Ctrl Pts',(36.2064052452609,-75.9999972411365,-79.4364776640188));
#30741=CARTESIAN_POINT('Ctrl Pts',(36.2050989509961,-75.9999982338138,-79.4357793353877));
#30742=CARTESIAN_POINT('Ctrl Pts',(36.2039708122481,-75.9999988737606,-79.4351762236091));
#30743=CARTESIAN_POINT('Ctrl Pts',(36.2028907204561,-75.9999994864524,-79.434598798108));
#30744=CARTESIAN_POINT('Ctrl Pts',(36.2019740763631,-75.9999997736227,-79.4341087287605));
#30745=CARTESIAN_POINT('Ctrl Pts',(36.2011210260212,-75.9999999102358,-79.4336526480419));
#30746=CARTESIAN_POINT('Ctrl Pts',(36.2007391952983,-75.9999999713846,-79.4334485034305));
#30747=CARTESIAN_POINT('Ctrl Pts',(36.2003695149134,-76.,-79.433250852737));
#30748=CARTESIAN_POINT('Ctrl Pts',(36.2,-76.,-79.4330532904862));
#30749=CARTESIAN_POINT('',(40.7249863758329,-74.3408331090314,-81.4672909116929));
#30750=CARTESIAN_POINT('Ctrl Pts',(40.7249863758336,-74.3408331090309,-81.467290911693));
#30751=CARTESIAN_POINT('Ctrl Pts',(40.2262052538249,-74.7634221949538,-81.3862769905682));
#30752=CARTESIAN_POINT('Ctrl Pts',(38.8816003633081,-75.6173708426798,-80.8780690735046));
#30753=CARTESIAN_POINT('Ctrl Pts',(37.2957669697243,-75.9669469406632,-80.0190459998239));
#30754=CARTESIAN_POINT('Ctrl Pts',(36.436575036449,-75.99600116153,-79.5595260981257));
#30755=CARTESIAN_POINT('',(41.0989794855664,-74.,-81.5));
#30756=CARTESIAN_POINT('Ctrl Pts',(41.0989794855664,-74.,-81.5));
#30757=CARTESIAN_POINT('Ctrl Pts',(40.9796542308205,-74.116914395022,-81.5));
#30758=CARTESIAN_POINT('Ctrl Pts',(40.8548672668006,-74.2307923625576,-81.4883866584888));
#30759=CARTESIAN_POINT('Ctrl Pts',(40.7249863758329,-74.3408331090314,-81.4672909116929));
#30760=CARTESIAN_POINT('',(41.2,-73.8989794855663,-81.5));
#30761=CARTESIAN_POINT('Origin',(36.2,-69.,-81.5));
#30762=CARTESIAN_POINT('',(41.5408331090314,-73.5249863758329,-81.4672909116929));
#30763=CARTESIAN_POINT('Ctrl Pts',(41.5408331090314,-73.5249863758329,-81.4672909116929));
#30764=CARTESIAN_POINT('Ctrl Pts',(41.4307923625576,-73.6548672668006,-81.4883866584888));
#30765=CARTESIAN_POINT('Ctrl Pts',(41.316914395022,-73.7796542308205,-81.5));
#30766=CARTESIAN_POINT('Ctrl Pts',(41.2,-73.8989794855663,-81.5));
#30767=CARTESIAN_POINT('',(43.196001093997,-69.2365770335277,-79.5595271661901));
#30768=CARTESIAN_POINT('Ctrl Pts',(43.196001093997,-69.2365770335277,-79.5595271661901));
#30769=CARTESIAN_POINT('Ctrl Pts',(43.1842694008473,-69.583503938841,-79.745073401727));
#30770=CARTESIAN_POINT('Ctrl Pts',(43.1462431487229,-69.9376909822518,-79.9350664222934));
#30771=CARTESIAN_POINT('Ctrl Pts',(43.0133707147083,-70.6455291845094,-80.3070714285095));
#30772=CARTESIAN_POINT('Ctrl Pts',(42.9185207631589,-70.9987198029951,-80.4888139716367));
#30773=CARTESIAN_POINT('Ctrl Pts',(42.6430856463133,-71.774189502708,-80.8664236862814));
#30774=CARTESIAN_POINT('Ctrl Pts',(42.4467748697811,-72.1911770437546,-81.0543062210682));
#30775=CARTESIAN_POINT('Ctrl Pts',(42.0361750904884,-72.8808297721556,-81.3118311224916));
#30776=CARTESIAN_POINT('Ctrl Pts',(41.8365825645193,-73.1647230633842,-81.398907956803));
#30777=CARTESIAN_POINT('Ctrl Pts',(41.5946015244113,-73.4609452952567,-81.4563646461124));
#30778=CARTESIAN_POINT('Ctrl Pts',(41.5678336290056,-73.4931177116952,-81.4621146824234));
#30779=CARTESIAN_POINT('Ctrl Pts',(41.5408331090314,-73.524986375833,-81.4672909116929));
#30780=CARTESIAN_POINT('Ctrl Pts',(43.2,-69.,-79.4330532904862));
#30781=CARTESIAN_POINT('Ctrl Pts',(43.2,-69.000829952749,-79.4334970271994));
#30782=CARTESIAN_POINT('Ctrl Pts',(43.1999998681034,-69.0016639948047,-79.4339429495971));
#30783=CARTESIAN_POINT('Ctrl Pts',(43.1999995080477,-69.002624372665,-79.4344563936532));
#30784=CARTESIAN_POINT('Ctrl Pts',(43.1999991342865,-69.0036213073114,-79.4349893819589));
#30785=CARTESIAN_POINT('Ctrl Pts',(43.1999985165435,-69.004754191808,-79.4355950302349));
#30786=CARTESIAN_POINT('Ctrl Pts',(43.199997334795,-69.0061084255198,-79.4363189799149));
#30787=CARTESIAN_POINT('Ctrl Pts',(43.1999960976964,-69.0075260882013,-79.4370768376138));
#30788=CARTESIAN_POINT('Ctrl Pts',(43.1999942436748,-69.0091860870021,-79.4379642132424));
#30789=CARTESIAN_POINT('Ctrl Pts',(43.1999911447523,-69.0111343338152,-79.4390056428645));
#30790=CARTESIAN_POINT('Ctrl Pts',(43.1999878573605,-69.0132010684564,-79.4401104098078));
#30791=CARTESIAN_POINT('Ctrl Pts',(43.1999831623473,-69.0155918671473,-79.4413883725242));
#30792=CARTESIAN_POINT('Ctrl Pts',(43.1999760573446,-69.0183083751824,-79.4428404081803));
#30793=CARTESIAN_POINT('Ctrl Pts',(43.1999683372839,-69.021260042912,-79.4444181420698));
#30794=CARTESIAN_POINT('Ctrl Pts',(43.1999577493602,-69.0245957858112,-79.4462011419664));
#30795=CARTESIAN_POINT('Ctrl Pts',(43.1999429445725,-69.0282625676438,-79.4481610611418));
#30796=CARTESIAN_POINT('Ctrl Pts',(43.199925558926,-69.0325685647166,-79.4504626450966));
#30797=CARTESIAN_POINT('Ctrl Pts',(43.1999022941867,-69.0373302706198,-79.45300777632));
#30798=CARTESIAN_POINT('Ctrl Pts',(43.1998716028295,-69.0423974515914,-79.4557161639972));
#30799=CARTESIAN_POINT('Ctrl Pts',(43.1998303537707,-69.0492077221319,-79.4593562259793));
#30800=CARTESIAN_POINT('Ctrl Pts',(43.1997754571138,-69.0565635915756,-79.463287874762));
#30801=CARTESIAN_POINT('Ctrl Pts',(43.1997070636227,-69.0640392338423,-79.4672835414457));
#30802=CARTESIAN_POINT('Ctrl Pts',(43.1996614454515,-69.0690254558109,-79.4699486343282));
#30803=CARTESIAN_POINT('Ctrl Pts',(43.1996099513757,-69.0740634750665,-79.4726414127713));
#30804=CARTESIAN_POINT('Ctrl Pts',(43.1995536343056,-69.0790501137166,-79.4753067390646));
#30805=CARTESIAN_POINT('Ctrl Pts',(43.1995030420523,-69.0835298440296,-79.4777011261113));
#30806=CARTESIAN_POINT('Ctrl Pts',(43.1994485978457,-69.0879675230588,-79.4800730453471));
#30807=CARTESIAN_POINT('Ctrl Pts',(43.1993911714285,-69.0923213373425,-79.4824001558459));
#30808=CARTESIAN_POINT('Ctrl Pts',(43.1993375274645,-69.0963883829329,-79.4845739886913));
#30809=CARTESIAN_POINT('Ctrl Pts',(43.1992813110251,-69.1003818731923,-79.4867085208521));
#30810=CARTESIAN_POINT('Ctrl Pts',(43.1992228530745,-69.1043046163885,-79.4888052625672));
#30811=CARTESIAN_POINT('Ctrl Pts',(43.1991663977533,-69.1080929757928,-79.4908301749301));
#30812=CARTESIAN_POINT('Ctrl Pts',(43.1991078793036,-69.1118149519592,-79.492819627487));
#30813=CARTESIAN_POINT('Ctrl Pts',(43.1990468225626,-69.1155143955378,-79.4947970718204));
#30814=CARTESIAN_POINT('Ctrl Pts',(43.1989837613951,-69.1193352878333,-79.4968394335048));
#30815=CARTESIAN_POINT('Ctrl Pts',(43.1989179008181,-69.1231385675992,-79.4988724198917));
#30816=CARTESIAN_POINT('Ctrl Pts',(43.1988478956635,-69.1269965880092,-79.5009347238157));
#30817=CARTESIAN_POINT('Ctrl Pts',(43.1987768113019,-69.1309140840829,-79.503028820442));
#30818=CARTESIAN_POINT('Ctrl Pts',(43.1987014292312,-69.1348878842858,-79.5051530722874));
#30819=CARTESIAN_POINT('Ctrl Pts',(43.1986209576208,-69.1389413241276,-79.5073199663836));
#30820=CARTESIAN_POINT('Ctrl Pts',(43.1985348423545,-69.1432790408708,-79.5096388296623));
#30821=CARTESIAN_POINT('Ctrl Pts',(43.198442875431,-69.1477075631141,-79.5120063144628));
#30822=CARTESIAN_POINT('Ctrl Pts',(43.1983451407054,-69.1522014834505,-79.5144088470743));
#30823=CARTESIAN_POINT('Ctrl Pts',(43.1982363478113,-69.1572038671642,-79.5170832135758));
#30824=CARTESIAN_POINT('Ctrl Pts',(43.1981203739986,-69.1622866610613,-79.5198006744928));
#30825=CARTESIAN_POINT('Ctrl Pts',(43.1979991016698,-69.1673576201683,-79.5225119144323));
#30826=CARTESIAN_POINT('Ctrl Pts',(43.1978294069763,-69.1744533431577,-79.5263057150058));
#30827=CARTESIAN_POINT('Ctrl Pts',(43.1976491625957,-69.1815242606409,-79.5300864654225));
#30828=CARTESIAN_POINT('Ctrl Pts',(43.197469069805,-69.1882195981374,-79.53366657499));
#30829=CARTESIAN_POINT('Ctrl Pts',(43.1973202003778,-69.193754139822,-79.5366259875136));
#30830=CARTESIAN_POINT('Ctrl Pts',(43.1971716764186,-69.1990271133279,-79.5394456619014));
#30831=CARTESIAN_POINT('Ctrl Pts',(43.1970312257634,-69.2038480455935,-79.5420236998639));
#30832=CARTESIAN_POINT('Ctrl Pts',(43.1969145600064,-69.2078525674018,-79.5441651548097));
#30833=CARTESIAN_POINT('Ctrl Pts',(43.1968035509037,-69.211544316003,-79.5461394170704));
#30834=CARTESIAN_POINT('Ctrl Pts',(43.1967020906367,-69.2148484463065,-79.5479064292267));
#30835=CARTESIAN_POINT('Ctrl Pts',(43.1966083302274,-69.217901824921,-79.5495393421672));
#30836=CARTESIAN_POINT('Ctrl Pts',(43.1965227694685,-69.2206235980485,-79.5509949530684));
#30837=CARTESIAN_POINT('Ctrl Pts',(43.1964471429847,-69.222996357416,-79.5522639279894));
#30838=CARTESIAN_POINT('Ctrl Pts',(43.1963784118337,-69.2251527776853,-79.5534172026444));
#30839=CARTESIAN_POINT('Ctrl Pts',(43.1963178969775,-69.227020852518,-79.5544162836341));
#30840=CARTESIAN_POINT('Ctrl Pts',(43.1962654046425,-69.2286271808036,-79.5552753829538));
#30841=CARTESIAN_POINT('Ctrl Pts',(43.1962147795399,-69.2301763695442,-79.5561039228016));
#30842=CARTESIAN_POINT('Ctrl Pts',(43.1961716280756,-69.2314817982239,-79.5568021000383));
#30843=CARTESIAN_POINT('Ctrl Pts',(43.1961341445413,-69.2326091820715,-79.5574050543386));
#30844=CARTESIAN_POINT('Ctrl Pts',(43.1960982574003,-69.2336885515516,-79.5579823293022));
#30845=CARTESIAN_POINT('Ctrl Pts',(43.1960675683624,-69.2346045746604,-79.5584722424537));
#30846=CARTESIAN_POINT('Ctrl Pts',(43.1960388775278,-69.235457053662,-79.5589281707014));
#30847=CARTESIAN_POINT('Ctrl Pts',(43.1960260388139,-69.235838525103,-79.5591321916864));
#30848=CARTESIAN_POINT('Ctrl Pts',(43.1960135779018,-69.2362078623941,-79.5593297231176));
#30849=CARTESIAN_POINT('Ctrl Pts',(43.196001093997,-69.2365770335277,-79.5595271661901));
#30850=CARTESIAN_POINT('Origin',(6.2,-74.,-12.));
#30851=CARTESIAN_POINT('Origin',(24.2,-74.,-66.));
#30852=CARTESIAN_POINT('Ctrl Pts',(-12.7511535426466,-68.7663011286799,
-80.439317485445));
#30853=CARTESIAN_POINT('Ctrl Pts',(-12.7518328402883,-68.7605155655161,
-80.436300501045));
#30854=CARTESIAN_POINT('Ctrl Pts',(-12.7531619882646,-68.7483736401701,
-80.429951673639));
#30855=CARTESIAN_POINT('Ctrl Pts',(-12.7616022324007,-68.6779765362022,
-80.3933108325196));
#30856=CARTESIAN_POINT('Ctrl Pts',(-12.7813230871559,-68.4664975829723,
-80.2821011164068));
#30857=CARTESIAN_POINT('Ctrl Pts',(-12.7946958959366,-68.2392841615299,
-80.1605544743685));
#30858=CARTESIAN_POINT('Ctrl Pts',(-12.8000922661796,-68.027860897069,-80.0472103201213));
#30859=CARTESIAN_POINT('Ctrl Pts',(-12.7998885602897,-67.9573139240965,
-80.009538072929));
#30860=CARTESIAN_POINT('Ctrl Pts',(-12.8,-67.9451437858327,-80.0030795017881));
#30861=CARTESIAN_POINT('Ctrl Pts',(-12.8,-67.9393398282202,-80.));
#30862=CARTESIAN_POINT('Ctrl Pts',(-12.7661027489825,-68.9230590967111,
-80.1460536890198));
#30863=CARTESIAN_POINT('Ctrl Pts',(-12.7664587807622,-68.9186438738067,
-80.1437379536791));
#30864=CARTESIAN_POINT('Ctrl Pts',(-12.7670812297361,-68.9106614644948,
-80.1395507592229));
#30865=CARTESIAN_POINT('Ctrl Pts',(-12.7731116474475,-68.8600406255686,
-80.1133008293174));
#30866=CARTESIAN_POINT('Ctrl Pts',(-12.7893842443182,-68.6893743987912,
-80.0237140866894));
#30867=CARTESIAN_POINT('Ctrl Pts',(-12.7981667187387,-68.5265712141199,
-79.9363677684688));
#30868=CARTESIAN_POINT('Ctrl Pts',(-12.8010845357288,-68.3560025283503,
-79.8447395802743));
#30869=CARTESIAN_POINT('Ctrl Pts',(-12.7999949300586,-68.3052975948829,
-79.8176043843904));
#30870=CARTESIAN_POINT('Ctrl Pts',(-12.8,-68.2973128834566,-79.8133650160724));
#30871=CARTESIAN_POINT('Ctrl Pts',(-12.8,-68.2928932188135,-79.8110177634954));
#30872=CARTESIAN_POINT('Ctrl Pts',(-12.7810519553184,-69.0798170647423,
-79.8527898925946));
#30873=CARTESIAN_POINT('Ctrl Pts',(-12.7811995792466,-69.0767879864804,
-79.8511897091324));
#30874=CARTESIAN_POINT('Ctrl Pts',(-12.7816990370264,-69.0691521434825,
-79.8471474801494));
#30875=CARTESIAN_POINT('Ctrl Pts',(-12.7844913839459,-69.0292068834798,
-79.8259370670281));
#30876=CARTESIAN_POINT('Ctrl Pts',(-12.7898784436764,-68.927771195494,-79.7719437530437));
#30877=CARTESIAN_POINT('Ctrl Pts',(-12.79660606409,-68.7983573463475,-79.7030234814484));
#30878=CARTESIAN_POINT('Ctrl Pts',(-12.7989499010098,-68.6970571314706,
-79.649006544579));
#30879=CARTESIAN_POINT('Ctrl Pts',(-12.7998185075757,-68.6571253855047,
-79.6277190371445));
#30880=CARTESIAN_POINT('Ctrl Pts',(-12.8,-68.6494819810805,-79.6236505303568));
#30881=CARTESIAN_POINT('Ctrl Pts',(-12.8,-68.6464466094067,-79.6220355269908));
#30882=CARTESIAN_POINT('Ctrl Pts',(-12.7960011616543,-69.2365750327735,
-79.5595260961694));
#30883=CARTESIAN_POINT('Ctrl Pts',(-12.7960569558779,-69.2349250849804,
-79.5586436579119));
#30884=CARTESIAN_POINT('Ctrl Pts',(-12.7961660004731,-69.2314614737188,
-79.5567913389998));
#30885=CARTESIAN_POINT('Ctrl Pts',(-12.796861884166,-69.2113439506909,-79.5460314217622));
#30886=CARTESIAN_POINT('Ctrl Pts',(-12.7984815301387,-69.1508161838819,
-79.513665787615));
#30887=CARTESIAN_POINT('Ctrl Pts',(-12.7995668885118,-69.0857768265977,
-79.4789020769686));
#30888=CARTESIAN_POINT('Ctrl Pts',(-12.8000074624845,-69.0252595353931,
-79.4465563372793));
#30889=CARTESIAN_POINT('Ctrl Pts',(-12.799990882671,-69.0051144027225,-79.4357877041059));
#30890=CARTESIAN_POINT('Ctrl Pts',(-12.8,-69.0016510787044,-79.4339360446411));
#30891=CARTESIAN_POINT('Ctrl Pts',(-12.8,-69.,-79.4330532904862));
#30892=CARTESIAN_POINT('',(-12.8,-67.9393398282202,-80.));
#30893=CARTESIAN_POINT('',(-12.7511535426466,-68.7663011286799,-80.439317485445));
#30894=CARTESIAN_POINT('Ctrl Pts',(-12.8,-67.9393398282202,-80.));
#30895=CARTESIAN_POINT('Ctrl Pts',(-12.8,-67.9414419655024,-80.0011153657472));
#30896=CARTESIAN_POINT('Ctrl Pts',(-12.7999991196284,-67.9435480069317,
-80.0022328244921));
#30897=CARTESIAN_POINT('Ctrl Pts',(-12.7999970367979,-67.9458263157412,
-80.0034427895298));
#30898=CARTESIAN_POINT('Ctrl Pts',(-12.7999949009835,-67.9481625810128,
-80.0046835341056));
#30899=CARTESIAN_POINT('Ctrl Pts',(-12.7999915030358,-67.95067986371,-80.0060214843292));
#30900=CARTESIAN_POINT('Ctrl Pts',(-12.7999858311703,-67.9535115086725,
-80.0075282878437));
#30901=CARTESIAN_POINT('Ctrl Pts',(-12.7999799943207,-67.9564255209836,
-80.0090789215036));
#30902=CARTESIAN_POINT('Ctrl Pts',(-12.7999717556751,-67.9596723045347,
-80.0108082974406));
#30903=CARTESIAN_POINT('Ctrl Pts',(-12.7999592405442,-67.9633488277327,
-80.0127685614673));
#30904=CARTESIAN_POINT('Ctrl Pts',(-12.799946040306,-67.9672266123404,-80.0148361348949));
#30905=CARTESIAN_POINT('Ctrl Pts',(-12.7999280866335,-67.9715824544212,
-80.0171605578629));
#30906=CARTESIAN_POINT('Ctrl Pts',(-12.7999022340551,-67.9764781077637,
-80.0197750909363));
#30907=CARTESIAN_POINT('Ctrl Pts',(-12.7998752238266,-67.9815929830961,
-80.0225066999344));
#30908=CARTESIAN_POINT('Ctrl Pts',(-12.7998395772213,-67.9872968847195,
-80.0255548709977));
#30909=CARTESIAN_POINT('Ctrl Pts',(-12.7997907696023,-67.9936068349789,
-80.0289288405153));
#30910=CARTESIAN_POINT('Ctrl Pts',(-12.7997391599796,-68.0002790340856,
-80.032496506737));
#30911=CARTESIAN_POINT('Ctrl Pts',(-12.7996727937154,-68.0076285898944,
-80.0364283082196));
#30912=CARTESIAN_POINT('Ctrl Pts',(-12.7995857188208,-68.0156208516721,
-80.0407056886438));
#30913=CARTESIAN_POINT('Ctrl Pts',(-12.799491696128,-68.0242508244868,-80.045324365785));
#30914=CARTESIAN_POINT('Ctrl Pts',(-12.7993734425619,-68.0336297662844,
-80.0503457624994));
#30915=CARTESIAN_POINT('Ctrl Pts',(-12.7992237895711,-68.04365689647,-80.0557156998772));
#30916=CARTESIAN_POINT('Ctrl Pts',(-12.7990546437389,-68.0549900965059,
-80.0617850909547));
#30917=CARTESIAN_POINT('Ctrl Pts',(-12.7988452033844,-68.0671506433314,
-80.0682993625326));
#30918=CARTESIAN_POINT('Ctrl Pts',(-12.7985877510598,-68.0799305652783,
-80.0751465322796));
#30919=CARTESIAN_POINT('Ctrl Pts',(-12.7982019864598,-68.0990799028725,
-80.0854062792165));
#30920=CARTESIAN_POINT('Ctrl Pts',(-12.7977069522051,-68.1196165458355,
-80.0964116800166));
#30921=CARTESIAN_POINT('Ctrl Pts',(-12.7970969250991,-68.1407215549374,
-80.1077212688361));
#30922=CARTESIAN_POINT('Ctrl Pts',(-12.7966664795798,-68.1556136089336,
-80.1157015073929));
#30923=CARTESIAN_POINT('Ctrl Pts',(-12.7961794307637,-68.170784726054,-80.1238310754694));
#30924=CARTESIAN_POINT('Ctrl Pts',(-12.7956415403645,-68.1859667653999,
-80.1319653074543));
#30925=CARTESIAN_POINT('Ctrl Pts',(-12.7951858474735,-68.1988287674205,
-80.1388565100024));
#30926=CARTESIAN_POINT('Ctrl Pts',(-12.7946938680268,-68.2116980075239,
-80.1457507392318));
#30927=CARTESIAN_POINT('Ctrl Pts',(-12.7941713799325,-68.2244477542231,
-80.1525795119216));
#30928=CARTESIAN_POINT('Ctrl Pts',(-12.7936920887942,-68.2361434094446,
-80.158843712525));
#30929=CARTESIAN_POINT('Ctrl Pts',(-12.7931872421108,-68.2477381387599,
-80.1650526367671));
#30930=CARTESIAN_POINT('Ctrl Pts',(-12.7926613499875,-68.2591736887779,
-80.1711746016963));
#30931=CARTESIAN_POINT('Ctrl Pts',(-12.7921657812218,-68.2699498558987,
-80.176943569265));
#30932=CARTESIAN_POINT('Ctrl Pts',(-12.7916516116072,-68.280584401439,-80.1826351780779));
#30933=CARTESIAN_POINT('Ctrl Pts',(-12.791121256113,-68.2910697963873,-80.1882449028664));
#30934=CARTESIAN_POINT('Ctrl Pts',(-12.7906144706368,-68.3010892002192,
-80.1936053206968));
#30935=CARTESIAN_POINT('Ctrl Pts',(-12.7900929767344,-68.3109722050848,
-80.1988908644493));
#30936=CARTESIAN_POINT('Ctrl Pts',(-12.7895564864506,-68.3207544709881,
-80.2041200314091));
#30937=CARTESIAN_POINT('Ctrl Pts',(-12.7890131201761,-68.3306621124503,
-80.209416218601));
#30938=CARTESIAN_POINT('Ctrl Pts',(-12.7884544756481,-68.3404657829456,
-80.2146542462203));
#30939=CARTESIAN_POINT('Ctrl Pts',(-12.7878764039241,-68.3502537016393,
-80.2198804282375));
#30940=CARTESIAN_POINT('Ctrl Pts',(-12.7873214743126,-68.3596497777528,
-80.2248973889983));
#30941=CARTESIAN_POINT('Ctrl Pts',(-12.7867481764485,-68.3690393498493,
-80.2299076786562));
#30942=CARTESIAN_POINT('Ctrl Pts',(-12.7861507958922,-68.3785104590878,
-80.2349574769543));
#30943=CARTESIAN_POINT('Ctrl Pts',(-12.7855161529563,-68.3885723409324,
-80.2403222629086));
#30944=CARTESIAN_POINT('Ctrl Pts',(-12.7848542677531,-68.3987262854919,
-80.2457316537937));
#30945=CARTESIAN_POINT('Ctrl Pts',(-12.7841604748655,-68.4090221920418,
-80.2512114845732));
#30946=CARTESIAN_POINT('Ctrl Pts',(-12.783443890586,-68.4196563235084,-80.2568713301285));
#30947=CARTESIAN_POINT('Ctrl Pts',(-12.7826932179844,-68.4304415244009,
-80.2626061141816));
#30948=CARTESIAN_POINT('Ctrl Pts',(-12.7819064372114,-68.4413782772843,
-80.2684154878918));
#30949=CARTESIAN_POINT('Ctrl Pts',(-12.7810713820932,-68.4529860742525,
-80.2745813061431));
#30950=CARTESIAN_POINT('Ctrl Pts',(-12.780195582854,-68.464764267707,-80.2808309643622));
#30951=CARTESIAN_POINT('Ctrl Pts',(-12.7792810579711,-68.4766581401074,
-80.2871349744576));
#30952=CARTESIAN_POINT('Ctrl Pts',(-12.7782865104577,-68.489592748495,-80.2939905971776));
#30953=CARTESIAN_POINT('Ctrl Pts',(-12.7772460715996,-68.502663678638,-80.300910220902));
#30954=CARTESIAN_POINT('Ctrl Pts',(-12.7761688047953,-68.5157431144594,
-80.3078260140958));
#30955=CARTESIAN_POINT('Ctrl Pts',(-12.7749095759397,-68.5310318088981,
-80.3159099597938));
#30956=CARTESIAN_POINT('Ctrl Pts',(-12.7735998467349,-68.5463312295996,
-80.3239881482717));
#30957=CARTESIAN_POINT('Ctrl Pts',(-12.7722651862118,-68.5613715074687,
-80.3319187178466));
#30958=CARTESIAN_POINT('Ctrl Pts',(-12.7705695625273,-68.5804794760765,
-80.3419941350561));
#30959=CARTESIAN_POINT('Ctrl Pts',(-12.7688336253202,-68.5991637065053,
-80.351828272569));
#30960=CARTESIAN_POINT('Ctrl Pts',(-12.7671305061878,-68.6168183625362,
-80.3611060393086));
#30961=CARTESIAN_POINT('Ctrl Pts',(-12.7659173876994,-68.6293936364735,
-80.3677145202709));
#30962=CARTESIAN_POINT('Ctrl Pts',(-12.7647215526255,-68.6414447795618,
-80.3740398914793));
#30963=CARTESIAN_POINT('Ctrl Pts',(-12.7635718386868,-68.6527752049831,
-80.3799810973145));
#30964=CARTESIAN_POINT('Ctrl Pts',(-12.7625391111644,-68.6629527298249,
-80.3853177698337));
#30965=CARTESIAN_POINT('Ctrl Pts',(-12.7615437904396,-68.6725480871623,
-80.3903441630596));
#30966=CARTESIAN_POINT('Ctrl Pts',(-12.7606047190396,-68.6814527914176,
-80.3950052350027));
#30967=CARTESIAN_POINT('Ctrl Pts',(-12.7597276128735,-68.6897699130019,
-80.3993587430981));
#30968=CARTESIAN_POINT('Ctrl Pts',(-12.758899695334,-68.6974841057397,-80.4033933523103));
#30969=CARTESIAN_POINT('Ctrl Pts',(-12.758132336613,-68.7045455229561,-80.4070844535359));
#30970=CARTESIAN_POINT('Ctrl Pts',(-12.7574026777113,-68.7112600174806,
-80.4105942134338));
#30971=CARTESIAN_POINT('Ctrl Pts',(-12.7567278489201,-68.7173839989792,
-80.4137932423359));
#30972=CARTESIAN_POINT('Ctrl Pts',(-12.7561125500973,-68.7229157499426,
-80.4166817626821));
#30973=CARTESIAN_POINT('Ctrl Pts',(-12.7554921827953,-68.7284930683007,
-80.4195940770039));
#30974=CARTESIAN_POINT('Ctrl Pts',(-12.7549324399538,-68.7334676634599,
-80.4221903926971));
#30975=CARTESIAN_POINT('Ctrl Pts',(-12.7544314042226,-68.7378886088854,
-80.4244972157607));
#30976=CARTESIAN_POINT('Ctrl Pts',(-12.753976436878,-68.7419030646919,-80.4265919349556));
#30977=CARTESIAN_POINT('Ctrl Pts',(-12.7535698402714,-68.7454612747732,
-80.4284480915835));
#30978=CARTESIAN_POINT('Ctrl Pts',(-12.7532043752489,-68.7486430334905,
-80.430107740582));
#30979=CARTESIAN_POINT('Ctrl Pts',(-12.7528471595585,-68.7517529730657,
-80.4317299277308));
#30980=CARTESIAN_POINT('Ctrl Pts',(-12.7525292584261,-68.7545030695974,
-80.4331642771879));
#30981=CARTESIAN_POINT('Ctrl Pts',(-12.7522381260796,-68.7570112163957,
-80.4344724376543));
#30982=CARTESIAN_POINT('Ctrl Pts',(-12.7519553737875,-68.7594471678263,
-80.435742943576));
#30983=CARTESIAN_POINT('Ctrl Pts',(-12.7516978784384,-68.7616547969803,
-80.4368943675231));
#30984=CARTESIAN_POINT('Ctrl Pts',(-12.7514484579662,-68.7637855518688,
-80.4380056117235));
#30985=CARTESIAN_POINT('Ctrl Pts',(-12.7513493910281,-68.7646318631635,
-80.4384469851179));
#30986=CARTESIAN_POINT('Ctrl Pts',(-12.7512515330953,-68.7654665461706,
-80.4388822776113));
#30987=CARTESIAN_POINT('Ctrl Pts',(-12.7511535426466,-68.7663011286799,
-80.439317485445));
#30988=CARTESIAN_POINT('',(-12.7960011616543,-69.2365750327735,-79.5595260961694));
#30989=CARTESIAN_POINT('Ctrl Pts',(-12.7960011616543,-69.2365750327735,
-79.5595260961694));
#30990=CARTESIAN_POINT('Ctrl Pts',(-12.7810519553184,-69.0798170647423,
-79.8527898925946));
#30991=CARTESIAN_POINT('Ctrl Pts',(-12.7661027489825,-68.9230590967111,
-80.1460536890198));
#30992=CARTESIAN_POINT('Ctrl Pts',(-12.7511535426466,-68.7663011286799,
-80.439317485445));
#30993=CARTESIAN_POINT('',(-12.8,-69.,-79.4330532904862));
#30994=CARTESIAN_POINT('Ctrl Pts',(-12.7960011616543,-69.2365750327735,
-79.5595260961694));
#30995=CARTESIAN_POINT('Ctrl Pts',(-12.7960292083229,-69.2357456361795,
-79.5590825116583));
#30996=CARTESIAN_POINT('Ctrl Pts',(-12.7960572613955,-69.2349121483207,
-79.5586367411658));
#30997=CARTESIAN_POINT('Ctrl Pts',(-12.7960893559361,-69.2339523963487,
-79.5581234407148));
#30998=CARTESIAN_POINT('Ctrl Pts',(-12.7961226721972,-69.2329561101666,
-79.557590600813));
#30999=CARTESIAN_POINT('Ctrl Pts',(-12.7961603390279,-69.2318239510054,
-79.5569850918275));
#31000=CARTESIAN_POINT('Ctrl Pts',(-12.7962049226453,-69.2304705628775,
-79.5562612669052));
#31001=CARTESIAN_POINT('Ctrl Pts',(-12.7962515945371,-69.229053782726,-79.5555035383852));
#31002=CARTESIAN_POINT('Ctrl Pts',(-12.7963058396059,-69.2273947972326,
-79.5546162755396));
#31003=CARTESIAN_POINT('Ctrl Pts',(-12.7963685818537,-69.2254477031397,
-79.5535749397574));
#31004=CARTESIAN_POINT('Ctrl Pts',(-12.7964351401458,-69.2233821848954,
-79.5524702689228));
#31005=CARTESIAN_POINT('Ctrl Pts',(-12.7965112434551,-69.2209927570776,
-79.5511923799426));
#31006=CARTESIAN_POINT('Ctrl Pts',(-12.7965959456592,-69.218277743219,-79.5497403965593));
#31007=CARTESIAN_POINT('Ctrl Pts',(-12.7966879808357,-69.2153276809137,
-79.5481627097886));
#31008=CARTESIAN_POINT('Ctrl Pts',(-12.7967901299217,-69.2119936833039,
-79.5463797291895));
#31009=CARTESIAN_POINT('Ctrl Pts',(-12.7968992523985,-69.2083287109004,
-79.5444198073676));
#31010=CARTESIAN_POINT('Ctrl Pts',(-12.7970274017946,-69.2040247030171,
-79.5421181477523));
#31011=CARTESIAN_POINT('Ctrl Pts',(-12.7971650772674,-69.1992650434548,
-79.5395728952846));
#31012=CARTESIAN_POINT('Ctrl Pts',(-12.7973056545457,-69.1941998374416,
-79.5368643629279));
#31013=CARTESIAN_POINT('Ctrl Pts',(-12.7974945510837,-69.1873936174649,
-79.5332248531063));
#31014=CARTESIAN_POINT('Ctrl Pts',(-12.7976882456695,-69.1800418837563,
-79.5292938348712));
#31015=CARTESIAN_POINT('Ctrl Pts',(-12.7978725057253,-69.172569967302,-79.5252987931617));
#31016=CARTESIAN_POINT('Ctrl Pts',(-12.797995425483,-69.1675854569241,-79.5226337035582));
#31017=CARTESIAN_POINT('Ctrl Pts',(-12.7981142248542,-69.1625489535661,
-79.5199409172442));
#31018=CARTESIAN_POINT('Ctrl Pts',(-12.7982264691812,-69.1575635936742,
-79.5172755781975));
#31019=CARTESIAN_POINT('Ctrl Pts',(-12.7983273034916,-69.1530850125295,
-79.5148811799079));
#31020=CARTESIAN_POINT('Ctrl Pts',(-12.7984228682132,-69.1486482922782,
-79.5125092455365));
#31021=CARTESIAN_POINT('Ctrl Pts',(-12.7985126194035,-69.144295239178,-79.5101821191301));
#31022=CARTESIAN_POINT('Ctrl Pts',(-12.7985964590319,-69.1402289047641,
-79.508008271494));
#31023=CARTESIAN_POINT('Ctrl Pts',(-12.7986752428822,-69.1362359540293,
-79.5058737238968));
#31024=CARTESIAN_POINT('Ctrl Pts',(-12.7987493965746,-69.1323135818703,
-79.5037769667935));
#31025=CARTESIAN_POINT('Ctrl Pts',(-12.7988210097945,-69.1285255884331,
-79.5017520436541));
#31026=CARTESIAN_POINT('Ctrl Pts',(-12.7988883185632,-69.1248038214923,
-79.4997625802429));
#31027=CARTESIAN_POINT('Ctrl Pts',(-12.7989523299241,-69.121104431999,-79.497785123555));
#31028=CARTESIAN_POINT('Ctrl Pts',(-12.7990184396467,-69.1172837725157,
-79.4957428436974));
#31029=CARTESIAN_POINT('Ctrl Pts',(-12.7990811576708,-69.1134805580376,
-79.4937099361942));
#31030=CARTESIAN_POINT('Ctrl Pts',(-12.799141584533,-69.1096224414086,-79.4916477126436));
#31031=CARTESIAN_POINT('Ctrl Pts',(-12.7992029440752,-69.1057047753016,
-79.4895536589676));
#31032=CARTESIAN_POINT('Ctrl Pts',(-12.7992619121947,-69.101730635701,-79.4874294505204));
#31033=CARTESIAN_POINT('Ctrl Pts',(-12.7993184858065,-69.0976766822073,
-79.4852626001243));
#31034=CARTESIAN_POINT('Ctrl Pts',(-12.799379027078,-69.0933384140429,-79.4829437826772));
#31035=CARTESIAN_POINT('Ctrl Pts',(-12.7994367896057,-69.088909139761,-79.4805763439809));
#31036=CARTESIAN_POINT('Ctrl Pts',(-12.7994909980303,-69.08441426712,-79.4781738549575));
#31037=CARTESIAN_POINT('Ctrl Pts',(-12.7995513398687,-69.0794108219781,
-79.4754995362408));
#31038=CARTESIAN_POINT('Ctrl Pts',(-12.7996072226821,-69.0743267169926,
-79.4727821199101));
#31039=CARTESIAN_POINT('Ctrl Pts',(-12.799657409628,-69.0692542261559,-79.4700709151347));
#31040=CARTESIAN_POINT('Ctrl Pts',(-12.7997276364042,-69.062156271242,-79.4662771164119));
#31041=CARTESIAN_POINT('Ctrl Pts',(-12.7997864800475,-69.055082683729,-79.4624963494086));
#31042=CARTESIAN_POINT('Ctrl Pts',(-12.7998327796974,-69.0483844631479,
-79.4589161926673));
#31043=CARTESIAN_POINT('Ctrl Pts',(-12.7998710512233,-69.0428476799647,
-79.455956816905));
#31044=CARTESIAN_POINT('Ctrl Pts',(-12.7999008268853,-69.0375723115798,
-79.4531371510512));
#31045=CARTESIAN_POINT('Ctrl Pts',(-12.7999233926443,-69.0327490016854,
-79.4505590809883));
#31046=CARTESIAN_POINT('Ctrl Pts',(-12.7999421370997,-69.0287424749182,
-79.4484175833567));
#31047=CARTESIAN_POINT('Ctrl Pts',(-12.7999559634565,-69.0250487403429,
-79.4464432528478));
#31048=CARTESIAN_POINT('Ctrl Pts',(-12.7999662322845,-69.0217427430679,
-79.4446761446091));
#31049=CARTESIAN_POINT('Ctrl Pts',(-12.7999757221325,-69.0186875344802,
-79.4430430869212));
#31050=CARTESIAN_POINT('Ctrl Pts',(-12.799982198985,-69.0159640572094,-79.4415873197681));
#31051=CARTESIAN_POINT('Ctrl Pts',(-12.7999868084143,-69.0135897765305,
-79.4403181795648));
#31052=CARTESIAN_POINT('Ctrl Pts',(-12.7999909974299,-69.0114320475654,
-79.4391647942041));
#31053=CARTESIAN_POINT('Ctrl Pts',(-12.7999936526088,-69.0095627953852,
-79.4381655843713));
#31054=CARTESIAN_POINT('Ctrl Pts',(-12.7999954793624,-69.007955432479,-79.4373063421029));
#31055=CARTESIAN_POINT('Ctrl Pts',(-12.7999972411368,-69.0064052448995,
-79.4364776638455));
#31056=CARTESIAN_POINT('Ctrl Pts',(-12.799998233814,-69.0050989506826,-79.4357793352319));
#31057=CARTESIAN_POINT('Ctrl Pts',(-12.7999988737608,-69.0039708119737,
-79.4351762234692));
#31058=CARTESIAN_POINT('Ctrl Pts',(-12.7999994864525,-69.002890720218,-79.434598797983));
#31059=CARTESIAN_POINT('Ctrl Pts',(-12.7999997736227,-69.0019740761535,
-79.4341087286492));
#31060=CARTESIAN_POINT('Ctrl Pts',(-12.7999999102358,-69.0011210258309,
-79.4336526479403));
#31061=CARTESIAN_POINT('Ctrl Pts',(-12.7999999713847,-69.0007391951752,
-79.4334485033647));
#31062=CARTESIAN_POINT('Ctrl Pts',(-12.8,-69.0003695148519,-79.4332508527041));
#31063=CARTESIAN_POINT('Ctrl Pts',(-12.8,-69.,-79.4330532904862));
#31064=CARTESIAN_POINT('',(-12.8,-68.4696699141101,-79.7165266452431));
#31065=CARTESIAN_POINT('Ctrl Pts',(-6.03657703353082,-75.9960010939969,
-79.5595271661918));
#31066=CARTESIAN_POINT('Ctrl Pts',(-6.03327711009717,-75.9961126843306,
-79.5577622746215));
#31067=CARTESIAN_POINT('Ctrl Pts',(-6.02026638500826,-75.996630632865,-79.5508024334891));
#31068=CARTESIAN_POINT('Ctrl Pts',(-5.95065337319764,-75.9985039356983,
-79.5135784929313));
#31069=CARTESIAN_POINT('Ctrl Pts',(-5.8859377473749,-75.9995834393596,-79.4789880070745));
#31070=CARTESIAN_POINT('Ctrl Pts',(-5.81635363943525,-76.0000779190584,
-79.4417961750041));
#31071=CARTESIAN_POINT('Ctrl Pts',(-5.80330218536736,-76.,-79.4348188137443));
#31072=CARTESIAN_POINT('Ctrl Pts',(-5.8,-76.,-79.4330532904862));
#31073=CARTESIAN_POINT('Ctrl Pts',(-5.87981905585798,-75.9810518330436,
-79.8527909486792));
#31074=CARTESIAN_POINT('Ctrl Pts',(-5.87376087109586,-75.9813470906745,
-79.8495905670206));
#31075=CARTESIAN_POINT('Ctrl Pts',(-5.84397742479736,-75.9831739264559,
-79.8337977365213));
#31076=CARTESIAN_POINT('Ctrl Pts',(-5.72771843298234,-75.9889126186106,
-79.7718564493927));
#31077=CARTESIAN_POINT('Ctrl Pts',(-5.59861589417875,-75.9951964527643,
-79.7031094075536));
#31078=CARTESIAN_POINT('Ctrl Pts',(-5.48236810616443,-75.9992414076862,
-79.6411504971624));
#31079=CARTESIAN_POINT('Ctrl Pts',(-5.45251738072014,-76.,-79.6252655486369));
#31080=CARTESIAN_POINT('Ctrl Pts',(-5.44644660940672,-76.,-79.6220355269908));
#31081=CARTESIAN_POINT('Ctrl Pts',(-5.72306107818513,-75.9661025720903,
-80.1460547311667));
#31082=CARTESIAN_POINT('Ctrl Pts',(-5.71423060572681,-75.9668146627209,
-80.141423247653));
#31083=CARTESIAN_POINT('Ctrl Pts',(-5.68537900484321,-75.9714758414277,
-80.1262751604081));
#31084=CARTESIAN_POINT('Ctrl Pts',(-5.48880129776891,-75.9845626296476,
-80.0204498936597));
#31085=CARTESIAN_POINT('Ctrl Pts',(-5.32713079429893,-75.9958857681933,
-79.9346800344166));
#31086=CARTESIAN_POINT('Ctrl Pts',(-5.13072552883509,-75.9990090085338,
-79.8304586573348));
#31087=CARTESIAN_POINT('Ctrl Pts',(-5.10173257607291,-76.,-79.8157122835296));
#31088=CARTESIAN_POINT('Ctrl Pts',(-5.09289321881345,-76.,-79.8110177634954));
#31089=CARTESIAN_POINT('Ctrl Pts',(-5.56630310051229,-75.9511533111369,
-80.4393185136542));
#31090=CARTESIAN_POINT('Ctrl Pts',(-5.55473194650397,-75.9525119129618,
-80.4332845306404));
#31091=CARTESIAN_POINT('Ctrl Pts',(-5.50914529119826,-75.9587873887317,
-80.4097053660028));
#31092=CARTESIAN_POINT('Ctrl Pts',(-5.26592447242786,-75.9815925202367,
-80.2818324443123));
#31093=CARTESIAN_POINT('Ctrl Pts',(-5.03984373668773,-75.994897210969,-80.1608657662782));
#31094=CARTESIAN_POINT('Ctrl Pts',(-4.79674752703822,-76.0009537785116,
-80.0305411221384));
#31095=CARTESIAN_POINT('Ctrl Pts',(-4.75094777142568,-76.,-80.0061590184222));
#31096=CARTESIAN_POINT('Ctrl Pts',(-4.73933982822017,-76.,-80.));
#31097=CARTESIAN_POINT('',(-5.8,-76.,-79.4330532904862));
#31098=CARTESIAN_POINT('',(-6.03657703353082,-75.9960010939969,-79.5595271661918));
#31099=CARTESIAN_POINT('Ctrl Pts',(-5.8,-76.,-79.4330532904862));
#31100=CARTESIAN_POINT('Ctrl Pts',(-5.80082995274897,-76.,-79.4334970271994));
#31101=CARTESIAN_POINT('Ctrl Pts',(-5.80166399480472,-75.9999998681034,
-79.4339429495971));
#31102=CARTESIAN_POINT('Ctrl Pts',(-5.80262437266497,-75.9999995080477,
-79.4344563936532));
#31103=CARTESIAN_POINT('Ctrl Pts',(-5.80362130731139,-75.9999991342865,
-79.4349893819589));
#31104=CARTESIAN_POINT('Ctrl Pts',(-5.80475419180803,-75.9999985165435,
-79.4355950302349));
#31105=CARTESIAN_POINT('Ctrl Pts',(-5.80610842551985,-75.999997334795,-79.4363189799149));
#31106=CARTESIAN_POINT('Ctrl Pts',(-5.80752608820132,-75.9999960976964,
-79.4370768376138));
#31107=CARTESIAN_POINT('Ctrl Pts',(-5.80918608700224,-75.9999942436748,
-79.4379642132424));
#31108=CARTESIAN_POINT('Ctrl Pts',(-5.8111343338153,-75.9999911447523,-79.4390056428645));
#31109=CARTESIAN_POINT('Ctrl Pts',(-5.81320106845652,-75.9999878573605,
-79.4401104098078));
#31110=CARTESIAN_POINT('Ctrl Pts',(-5.81559186714737,-75.9999831623473,
-79.4413883725241));
#31111=CARTESIAN_POINT('Ctrl Pts',(-5.81830837518257,-75.9999760573446,
-79.4428404081802));
#31112=CARTESIAN_POINT('Ctrl Pts',(-5.82126004291222,-75.9999683372839,
-79.4444181420697));
#31113=CARTESIAN_POINT('Ctrl Pts',(-5.82459578581144,-75.9999577493602,
-79.4462011419664));
#31114=CARTESIAN_POINT('Ctrl Pts',(-5.8282625676441,-75.9999429445725,-79.4481610611416));
#31115=CARTESIAN_POINT('Ctrl Pts',(-5.83256856471686,-75.999925558926,-79.4504626450964));
#31116=CARTESIAN_POINT('Ctrl Pts',(-5.8373302706201,-75.9999022941867,-79.4530077763197));
#31117=CARTESIAN_POINT('Ctrl Pts',(-5.84239745159174,-75.9998716028295,
-79.455716163997));
#31118=CARTESIAN_POINT('Ctrl Pts',(-5.84920772213249,-75.9998303537706,
-79.459356225979));
#31119=CARTESIAN_POINT('Ctrl Pts',(-5.85656359157639,-75.9997754571138,
-79.4632878747617));
#31120=CARTESIAN_POINT('Ctrl Pts',(-5.86403923384336,-75.9997070636227,
-79.4672835414454));
#31121=CARTESIAN_POINT('Ctrl Pts',(-5.86902545581198,-75.9996614454515,
-79.4699486343278));
#31122=CARTESIAN_POINT('Ctrl Pts',(-5.87406347506768,-75.9996099513757,
-79.4726414127709));
#31123=CARTESIAN_POINT('Ctrl Pts',(-5.87905011371789,-75.9995536343056,
-79.4753067390642));
#31124=CARTESIAN_POINT('Ctrl Pts',(-5.88352984403094,-75.9995030420523,
-79.4777011261108));
#31125=CARTESIAN_POINT('Ctrl Pts',(-5.88796752306019,-75.9994485978456,
-79.4800730453466));
#31126=CARTESIAN_POINT('Ctrl Pts',(-5.89232133734403,-75.9993911714285,
-79.4824001558454));
#31127=CARTESIAN_POINT('Ctrl Pts',(-5.89638838293447,-75.9993375274645,
-79.4845739886907));
#31128=CARTESIAN_POINT('Ctrl Pts',(-5.90038187319399,-75.9992813110251,
-79.4867085208515));
#31129=CARTESIAN_POINT('Ctrl Pts',(-5.90430461639031,-75.9992228530745,
-79.4888052625665));
#31130=CARTESIAN_POINT('Ctrl Pts',(-5.90809297579459,-75.9991663977532,
-79.4908301749294));
#31131=CARTESIAN_POINT('Ctrl Pts',(-5.91181495196092,-75.9991078793035,
-79.4928196274862));
#31132=CARTESIAN_POINT('Ctrl Pts',(-5.91551439553953,-75.9990468225626,
-79.4947970718196));
#31133=CARTESIAN_POINT('Ctrl Pts',(-5.91933528783517,-75.9989837613951,
-79.496839433504));
#31134=CARTESIAN_POINT('Ctrl Pts',(-5.92313856760111,-75.9989179008181,
-79.4988724198909));
#31135=CARTESIAN_POINT('Ctrl Pts',(-5.92699658801122,-75.9988478956635,
-79.5009347238149));
#31136=CARTESIAN_POINT('Ctrl Pts',(-5.93091408408494,-75.9987768113019,
-79.5030288204412));
#31137=CARTESIAN_POINT('Ctrl Pts',(-5.9348878842878,-75.9987014292312,-79.5051530722866));
#31138=CARTESIAN_POINT('Ctrl Pts',(-5.93894132412967,-75.9986209576208,
-79.5073199663828));
#31139=CARTESIAN_POINT('Ctrl Pts',(-5.94327904087287,-75.9985348423544,
-79.5096388296616));
#31140=CARTESIAN_POINT('Ctrl Pts',(-5.94770756311628,-75.998442875431,-79.5120063144621));
#31141=CARTESIAN_POINT('Ctrl Pts',(-5.95220148345265,-75.9983451407054,
-79.5144088470737));
#31142=CARTESIAN_POINT('Ctrl Pts',(-5.95720386716646,-75.9982363478113,
-79.5170832135752));
#31143=CARTESIAN_POINT('Ctrl Pts',(-5.96228666106351,-75.9981203739986,
-79.5198006744923));
#31144=CARTESIAN_POINT('Ctrl Pts',(-5.96735762017057,-75.9979991016698,
-79.5225119144319));
#31145=CARTESIAN_POINT('Ctrl Pts',(-5.97445334315968,-75.9978294069763,
-79.5263057150053));
#31146=CARTESIAN_POINT('Ctrl Pts',(-5.98152426064256,-75.9976491625957,
-79.530086465422));
#31147=CARTESIAN_POINT('Ctrl Pts',(-5.98821959813878,-75.9974690698049,
-79.5336665749896));
#31148=CARTESIAN_POINT('Ctrl Pts',(-5.99375413982361,-75.9973202003778,
-79.5366259875134));
#31149=CARTESIAN_POINT('Ctrl Pts',(-5.99902711332963,-75.9971716764186,
-79.5394456619015));
#31150=CARTESIAN_POINT('Ctrl Pts',(-6.0038480455955,-75.9970312257633,-79.5420236998642));
#31151=CARTESIAN_POINT('Ctrl Pts',(-6.00785256740384,-75.9969145600064,
-79.5441651548101));
#31152=CARTESIAN_POINT('Ctrl Pts',(-6.01154431600515,-75.9968035509036,
-79.546139417071));
#31153=CARTESIAN_POINT('Ctrl Pts',(-6.01484844630879,-75.9967020906366,
-79.5479064292275));
#31154=CARTESIAN_POINT('Ctrl Pts',(-6.01790182492339,-75.9966083302274,
-79.5495393421681));
#31155=CARTESIAN_POINT('Ctrl Pts',(-6.02062359805108,-75.9965227694684,
-79.5509949530694));
#31156=CARTESIAN_POINT('Ctrl Pts',(-6.02299635741864,-75.9964471429846,
-79.5522639279905));
#31157=CARTESIAN_POINT('Ctrl Pts',(-6.02515277768795,-75.9963784118336,
-79.5534172026455));
#31158=CARTESIAN_POINT('Ctrl Pts',(-6.02702085252075,-75.9963178969774,
-79.5544162836354));
#31159=CARTESIAN_POINT('Ctrl Pts',(-6.02862718080636,-75.9962654046424,
-79.5552753829552));
#31160=CARTESIAN_POINT('Ctrl Pts',(-6.03017636954699,-75.9962147795398,
-79.556103922803));
#31161=CARTESIAN_POINT('Ctrl Pts',(-6.03148179822677,-75.9961716280755,
-79.5568021000397));
#31162=CARTESIAN_POINT('Ctrl Pts',(-6.0326091820744,-75.9961341445412,-79.5574050543401));
#31163=CARTESIAN_POINT('Ctrl Pts',(-6.03368855155447,-75.9960982574002,
-79.5579823293037));
#31164=CARTESIAN_POINT('Ctrl Pts',(-6.03460457466333,-75.9960675683623,
-79.5584722424552));
#31165=CARTESIAN_POINT('Ctrl Pts',(-6.03545705366498,-75.9960388775277,
-79.5589281707029));
#31166=CARTESIAN_POINT('Ctrl Pts',(-6.03583852510599,-75.9960260388138,
-79.559132191688));
#31167=CARTESIAN_POINT('Ctrl Pts',(-6.03620786239713,-75.9960135779017,
-79.5593297231193));
#31168=CARTESIAN_POINT('Ctrl Pts',(-6.03657703353082,-75.9960010939969,
-79.5595271661918));
#31169=CARTESIAN_POINT('',(-5.56630310051229,-75.9511533111369,-80.4393185136542));
#31170=CARTESIAN_POINT('Ctrl Pts',(-5.56630310051229,-75.9511533111369,
-80.4393185136542));
#31171=CARTESIAN_POINT('Ctrl Pts',(-5.72306107818513,-75.9661025720903,
-80.1460547311667));
#31172=CARTESIAN_POINT('Ctrl Pts',(-5.87981905585798,-75.9810518330436,
-79.8527909486792));
#31173=CARTESIAN_POINT('Ctrl Pts',(-6.03657703353082,-75.9960010939969,
-79.5595271661918));
#31174=CARTESIAN_POINT('',(-4.73933982822017,-76.,-80.));
#31175=CARTESIAN_POINT('Ctrl Pts',(-5.56630310051229,-75.9511533111369,
-80.4393185136542));
#31176=CARTESIAN_POINT('Ctrl Pts',(-5.56420681552843,-75.9513994418688,
-80.4382253687547));
#31177=CARTESIAN_POINT('Ctrl Pts',(-5.56210662013596,-75.9516451623633,
-80.4371299982174));
#31178=CARTESIAN_POINT('Ctrl Pts',(-5.55983393131473,-75.9519098993802,
-80.4359446578429));
#31179=CARTESIAN_POINT('Ctrl Pts',(-5.55750339571347,-75.952181374752,-80.4347291469833));
#31180=CARTESIAN_POINT('Ctrl Pts',(-5.55499160002995,-75.9524728344429,
-80.4334190935274));
#31181=CARTESIAN_POINT('Ctrl Pts',(-5.55216503325917,-75.9527989364359,
-80.4319448041763));
#31182=CARTESIAN_POINT('Ctrl Pts',(-5.54925619217981,-75.9531345304445,
-80.4304276019394));
#31183=CARTESIAN_POINT('Ctrl Pts',(-5.54601413463847,-75.9535068018879,
-80.428736540034));
#31184=CARTESIAN_POINT('Ctrl Pts',(-5.54234178307442,-75.9539253137786,
-80.4268206510647));
#31185=CARTESIAN_POINT('Ctrl Pts',(-5.53846827069886,-75.9543667505418,
-80.4247998152314));
#31186=CARTESIAN_POINT('Ctrl Pts',(-5.53411605254984,-75.9548596340652,
-80.4225288569658));
#31187=CARTESIAN_POINT('Ctrl Pts',(-5.52922332488371,-75.9554081743592,
-80.4199748464482));
#31188=CARTESIAN_POINT('Ctrl Pts',(-5.52411129332526,-75.9559813015565,
-80.4173063589996));
#31189=CARTESIAN_POINT('Ctrl Pts',(-5.51840942455183,-75.9566151484006,
-80.414328981764));
#31190=CARTESIAN_POINT('Ctrl Pts',(-5.51210072583542,-75.9573073476311,
-80.4110327808206));
#31191=CARTESIAN_POINT('Ctrl Pts',(-5.50542940200128,-75.9580393345958,
-80.4075471136642));
#31192=CARTESIAN_POINT('Ctrl Pts',(-5.49807975731088,-75.9588365034254,
-80.4037050492189));
#31193=CARTESIAN_POINT('Ctrl Pts',(-5.49008657713406,-75.9596890414977,
-80.399523291729));
#31194=CARTESIAN_POINT('Ctrl Pts',(-5.48145450988579,-75.9606097221039,
-80.395007290454));
#31195=CARTESIAN_POINT('Ctrl Pts',(-5.47207231574455,-75.9615948484974,
-80.39009530727));
#31196=CARTESIAN_POINT('Ctrl Pts',(-5.46204108178782,-75.962625655139,-80.3848383268206));
#31197=CARTESIAN_POINT('Ctrl Pts',(-5.45069945656391,-75.9637911172006,
-80.3788946211584));
#31198=CARTESIAN_POINT('Ctrl Pts',(-5.43852884548578,-75.9650147154232,
-80.3725102190935));
#31199=CARTESIAN_POINT('Ctrl Pts',(-5.42573797772755,-75.9662645146503,
-80.3657920972725));
#31200=CARTESIAN_POINT('Ctrl Pts',(-5.40663505197305,-75.9681310668103,
-80.3557587058889));
#31201=CARTESIAN_POINT('Ctrl Pts',(-5.38615199235454,-75.9700542679493,
-80.3449823921339));
#31202=CARTESIAN_POINT('Ctrl Pts',(-5.36510219960243,-75.9719331684186,
-80.3338855781411));
#31203=CARTESIAN_POINT('Ctrl Pts',(-5.35021359138999,-75.9732621227359,
-80.3260367542647));
#31204=CARTESIAN_POINT('Ctrl Pts',(-5.33504537194617,-75.9745690761541,
-80.3180297742239));
#31205=CARTESIAN_POINT('Ctrl Pts',(-5.31986575382764,-75.9758280745175,
-80.3100055159971));
#31206=CARTESIAN_POINT('Ctrl Pts',(-5.30700487317325,-75.9768947566678,
-80.3032069900665));
#31207=CARTESIAN_POINT('Ctrl Pts',(-5.29413641239381,-75.9779271418622,
-80.2963964149645));
#31208=CARTESIAN_POINT('Ctrl Pts',(-5.28138714940104,-75.9789158885675,
-80.2896409949838));
#31209=CARTESIAN_POINT('Ctrl Pts',(-5.26969165141048,-75.9798229123782,
-80.2834439308198));
#31210=CARTESIAN_POINT('Ctrl Pts',(-5.25809683612155,-75.9806932835307,
-80.2772934958828));
#31211=CARTESIAN_POINT('Ctrl Pts',(-5.24666095829357,-75.9815244583872,
-80.2712209815137));
#31212=CARTESIAN_POINT('Ctrl Pts',(-5.23588434009871,-75.9823077173742,
-80.2654985376555));
#31213=CARTESIAN_POINT('Ctrl Pts',(-5.22524913290962,-75.9830562233904,
-80.2598454426357));
#31214=CARTESIAN_POINT('Ctrl Pts',(-5.21476282203278,-75.9837713308532,
-80.2542662126294));
#31215=CARTESIAN_POINT('Ctrl Pts',(-5.20474245968912,-75.9844546632449,
-80.2489348900205));
#31216=CARTESIAN_POINT('Ctrl Pts',(-5.19485826674047,-75.9851075444798,
-80.2436711326451));
#31217=CARTESIAN_POINT('Ctrl Pts',(-5.18507449508653,-75.9857337373977,
-80.2384565456445));
#31218=CARTESIAN_POINT('Ctrl Pts',(-5.17521478296077,-75.9863647907505,
-80.2332014836398));
#31219=CARTESIAN_POINT('Ctrl Pts',(-5.16545763849053,-75.9869687713007,
-80.2279966720334));
#31220=CARTESIAN_POINT('Ctrl Pts',(-5.15571614445803,-75.9875516791372,
-80.2227965950344));
#31221=CARTESIAN_POINT('Ctrl Pts',(-5.14631664806357,-75.9881141226484,
-80.2177790787437));
#31222=CARTESIAN_POINT('Ctrl Pts',(-5.13692376966904,-75.9886574246325,
-80.2127617589355));
#31223=CARTESIAN_POINT('Ctrl Pts',(-5.12744922457989,-75.9891861239043,
-80.2076982534025));
#31224=CARTESIAN_POINT('Ctrl Pts',(-5.11738549871931,-75.9897477006856,
-80.2023198704724));
#31225=CARTESIAN_POINT('Ctrl Pts',(-5.10722959513758,-75.9902927448358,
-80.1968893513437));
#31226=CARTESIAN_POINT('Ctrl Pts',(-5.09693143911862,-75.9908223093185,
-80.1913805965077));
#31227=CARTESIAN_POINT('Ctrl Pts',(-5.08630134840889,-75.9913689429565,
-80.1856942810648));
#31228=CARTESIAN_POINT('Ctrl Pts',(-5.07552006464755,-75.9918989882314,
-80.1799247984738));
#31229=CARTESIAN_POINT('Ctrl Pts',(-5.06458696526359,-75.9924103020835,
-80.1740723646978));
#31230=CARTESIAN_POINT('Ctrl Pts',(-5.05298361295765,-75.992952961997,-80.1678611478631));
#31231=CARTESIAN_POINT('Ctrl Pts',(-5.04120958294207,-75.9934744148136,
-80.1615566624296));
#31232=CARTESIAN_POINT('Ctrl Pts',(-5.0293193642881,-75.9939700334766,-80.1551886129752));
#31233=CARTESIAN_POINT('Ctrl Pts',(-5.01639002675629,-75.9945089656164,
-80.148264042182));
#31234=CARTESIAN_POINT('Ctrl Pts',(-5.0033237905166,-75.9950171983507,-80.1412645651398));
#31235=CARTESIAN_POINT('Ctrl Pts',(-4.99024809552006,-75.9954885369991,
-80.1342590730832));
#31236=CARTESIAN_POINT('Ctrl Pts',(-4.97497270795401,-75.9960391678093,
-80.1260750640279));
#31237=CARTESIAN_POINT('Ctrl Pts',(-4.95968530337708,-75.9965391539293,
-80.1178833208327));
#31238=CARTESIAN_POINT('Ctrl Pts',(-4.94465465779552,-75.9969821282777,
-80.1098288638723));
#31239=CARTESIAN_POINT('Ctrl Pts',(-4.9255177507954,-75.9975461199481,-80.0995739887274));
#31240=CARTESIAN_POINT('Ctrl Pts',(-4.90680250399691,-75.9980169438008,
-80.0895446021287));
#31241=CARTESIAN_POINT('Ctrl Pts',(-4.88911665148895,-75.9983966220755,
-80.0800683512843));
#31242=CARTESIAN_POINT('Ctrl Pts',(-4.87653281631635,-75.9986667707055,
-80.0733258106786));
#31243=CARTESIAN_POINT('Ctrl Pts',(-4.86447189641292,-75.9988912194174,
-80.066864252552));
#31244=CARTESIAN_POINT('Ctrl Pts',(-4.85313058056598,-75.9990759421802,
-80.0607896158592));
#31245=CARTESIAN_POINT('Ctrl Pts',(-4.84294408761826,-75.999241855655,-80.0553335255195));
#31246=CARTESIAN_POINT('Ctrl Pts',(-4.83333877115914,-75.999375843044,-80.0501899245532));
#31247=CARTESIAN_POINT('Ctrl Pts',(-4.8244232494793,-75.9994842520891,-80.0454172395432));
#31248=CARTESIAN_POINT('Ctrl Pts',(-4.81609630495915,-75.99958550428,-80.0409596335031));
#31249=CARTESIAN_POINT('Ctrl Pts',(-4.80837149988448,-75.99966451597,-80.0368258070939));
#31250=CARTESIAN_POINT('Ctrl Pts',(-4.80129886613601,-75.9997270278736,
-80.0330426087309));
#31251=CARTESIAN_POINT('Ctrl Pts',(-4.79457383079584,-75.9997864675076,
-80.0294453430454));
#31252=CARTESIAN_POINT('Ctrl Pts',(-4.78843874020103,-75.9998310313963,
-80.0261652479022));
#31253=CARTESIAN_POINT('Ctrl Pts',(-4.78289555168418,-75.9998653972212,
-80.0232032971218));
#31254=CARTESIAN_POINT('Ctrl Pts',(-4.77729879020271,-75.9999000951797,
-80.0202127201302));
#31255=CARTESIAN_POINT('Ctrl Pts',(-4.77230613724924,-75.9999244270673,
-80.0175468458571));
#31256=CARTESIAN_POINT('Ctrl Pts',(-4.76786861194713,-75.9999423966778,
-80.0151792611979));
#31257=CARTESIAN_POINT('Ctrl Pts',(-4.76384513769839,-75.9999586896025,
-80.0130325881629));
#31258=CARTESIAN_POINT('Ctrl Pts',(-4.76027774664032,-75.9999697470085,
-80.0111309831632));
#31259=CARTESIAN_POINT('Ctrl Pts',(-4.75708692753788,-75.9999777607848,
-80.0094316682683));
#31260=CARTESIAN_POINT('Ctrl Pts',(-4.75396812364608,-75.9999855936941,
-80.007770706071));
#31261=CARTESIAN_POINT('Ctrl Pts',(-4.7512092797227,-75.9999905148514,-80.0063031091167));
#31262=CARTESIAN_POINT('Ctrl Pts',(-4.74869284463608,-75.9999938354518,
-80.0049656978208));
#31263=CARTESIAN_POINT('Ctrl Pts',(-4.74624891473313,-75.9999970603769,
-80.0036668208992));
#31264=CARTESIAN_POINT('Ctrl Pts',(-4.74403372650234,-75.9999987706602,
-80.0024907890072));
#31265=CARTESIAN_POINT('Ctrl Pts',(-4.74189623642452,-75.9999995399948,
-80.0013564736068));
#31266=CARTESIAN_POINT('Ctrl Pts',(-4.74103601494663,-75.9999998496094,
-80.0008999744256));
#31267=CARTESIAN_POINT('Ctrl Pts',(-4.74018786870459,-76.,-80.0004499588664));
#31268=CARTESIAN_POINT('Ctrl Pts',(-4.73933982822017,-76.,-80.));
#31269=CARTESIAN_POINT('',(-5.26966991411008,-76.,-79.7165266452431));
#31270=CARTESIAN_POINT('Ctrl Pts',(-5.56630310051229,-75.9511533111369,
-80.4393185136542));
#31271=CARTESIAN_POINT('Ctrl Pts',(-6.42601048595868,-75.8502126424846,
-80.8876281426549));
#31272=CARTESIAN_POINT('Ctrl Pts',(-8.03268023872916,-75.3730832556622,
-81.6648999492777));
#31273=CARTESIAN_POINT('Ctrl Pts',(-9.43111245203295,-74.4444873881411,
-82.0000000010328));
#31274=CARTESIAN_POINT('Ctrl Pts',(-9.95543453132142,-73.9999999953529,
-82.));
#31275=CARTESIAN_POINT('Ctrl Pts',(-5.72306107818513,-75.9661025720903,
-80.1460547311667));
#31276=CARTESIAN_POINT('Ctrl Pts',(-6.58258916750901,-75.8891242237522,
-80.5980971288505));
#31277=CARTESIAN_POINT('Ctrl Pts',(-8.18232324202342,-75.4545140008688,
-81.4026226152872));
#31278=CARTESIAN_POINT('Ctrl Pts',(-9.56281012582098,-74.5507989284016,
-81.7954256760992));
#31279=CARTESIAN_POINT('Ctrl Pts',(-10.0786184794921,-74.1136110332455,
-81.8224303038977));
#31280=CARTESIAN_POINT('Ctrl Pts',(-5.87981905585798,-75.9810518330436,
-79.8527909486792));
#31281=CARTESIAN_POINT('Ctrl Pts',(-6.73916784905935,-75.9280358050199,
-80.3085661150462));
#31282=CARTESIAN_POINT('Ctrl Pts',(-8.33196624531768,-75.5359447460753,
-81.1403452812968));
#31283=CARTESIAN_POINT('Ctrl Pts',(-9.69450779960901,-74.6571104686622,
-81.5908513511656));
#31284=CARTESIAN_POINT('Ctrl Pts',(-10.2018024276628,-74.2272220711382,
-81.6448606077953));
#31285=CARTESIAN_POINT('Ctrl Pts',(-6.03657703353082,-75.9960010939969,
-79.5595271661918));
#31286=CARTESIAN_POINT('Ctrl Pts',(-6.89574653060969,-75.9669473862876,
-80.0190351012419));
#31287=CARTESIAN_POINT('Ctrl Pts',(-8.48160924861194,-75.6173754912818,
-80.8780679473063));
#31288=CARTESIAN_POINT('Ctrl Pts',(-9.82620547339704,-74.7634220089227,
-81.386277026232));
#31289=CARTESIAN_POINT('Ctrl Pts',(-10.3249863758336,-74.3408331090309,
-81.467290911693));
#31290=CARTESIAN_POINT('',(-10.3249863758329,-74.3408331090314,-81.4672909116929));
#31291=CARTESIAN_POINT('Ctrl Pts',(-6.03657703353082,-75.9960010939969,
-79.5595271661918));
#31292=CARTESIAN_POINT('Ctrl Pts',(-6.89574653060969,-75.9669473862876,
-80.0190351012419));
#31293=CARTESIAN_POINT('Ctrl Pts',(-8.48160924861194,-75.6173754912818,
-80.8780679473063));
#31294=CARTESIAN_POINT('Ctrl Pts',(-9.82620547339704,-74.7634220089227,
-81.386277026232));
#31295=CARTESIAN_POINT('Ctrl Pts',(-10.3249863758336,-74.3408331090309,
-81.467290911693));
#31296=CARTESIAN_POINT('',(-10.3249863758329,-74.3408331090314,-81.4672909116929));
#31297=CARTESIAN_POINT('Ctrl Pts',(-9.95543453132142,-73.9999999953529,
-82.));
#31298=CARTESIAN_POINT('Ctrl Pts',(-9.43111245203295,-74.4444873881411,
-82.0000000010328));
#31299=CARTESIAN_POINT('Ctrl Pts',(-8.03268023872916,-75.3730832556622,
-81.6648999492777));
#31300=CARTESIAN_POINT('Ctrl Pts',(-6.42601048595868,-75.8502126424846,
-80.8876281426549));
#31301=CARTESIAN_POINT('Ctrl Pts',(-5.56630310051229,-75.9511533111369,
-80.4393185136542));
#31302=CARTESIAN_POINT('Origin',(-5.8,-69.,-81.75));
#31303=CARTESIAN_POINT('',(-10.6989794855664,-74.,-81.5));
#31304=CARTESIAN_POINT('',(-10.3490523794545,-73.6428571428571,-82.));
#31305=CARTESIAN_POINT('',(-10.8,-73.8989794855664,-81.5));
#31306=CARTESIAN_POINT('Origin',(-5.8,-69.,-81.5));
#31307=CARTESIAN_POINT('',(-10.8,-73.8989794855664,-81.5));
#31308=CARTESIAN_POINT('Ctrl Pts',(-9.95543453132077,-73.9999999953534,
-82.));
#31309=CARTESIAN_POINT('Ctrl Pts',(-10.0919662599274,-73.8842569540723,
-82.));
#31310=CARTESIAN_POINT('Ctrl Pts',(-10.2227896098978,-73.7665688864269,
-82.));
#31311=CARTESIAN_POINT('Ctrl Pts',(-10.3490523794545,-73.6428571428571,
-82.));
#31312=CARTESIAN_POINT('Ctrl Pts',(-10.0786184794915,-74.1136110332461,
-81.8224303038976));
#31313=CARTESIAN_POINT('Ctrl Pts',(-10.2129332622185,-73.9997687569007,
-81.8294622194963));
#31314=CARTESIAN_POINT('Ctrl Pts',(-10.3417444835387,-73.8833507226252,
-81.8333333333333));
#31315=CARTESIAN_POINT('Ctrl Pts',(-10.4656947481584,-73.7619047619048,
-81.8333333333333));
#31316=CARTESIAN_POINT('Ctrl Pts',(-10.2018024276622,-74.2272220711388,
-81.6448606077953));
#31317=CARTESIAN_POINT('Ctrl Pts',(-10.3339002645095,-74.1152805597292,
-81.6589244389925));
#31318=CARTESIAN_POINT('Ctrl Pts',(-10.4606993571796,-74.0001325588236,
-81.6666666666667));
#31319=CARTESIAN_POINT('Ctrl Pts',(-10.5823371168624,-73.8809523809524,
-81.6666666666667));
#31320=CARTESIAN_POINT('Ctrl Pts',(-10.3249863758329,-74.3408331090314,
-81.4672909116929));
#31321=CARTESIAN_POINT('Ctrl Pts',(-10.4548672668006,-74.2307923625576,
-81.4883866584888));
#31322=CARTESIAN_POINT('Ctrl Pts',(-10.5796542308205,-74.116914395022,-81.5));
#31323=CARTESIAN_POINT('Ctrl Pts',(-10.6989794855664,-74.,-81.5));
#31324=CARTESIAN_POINT('Ctrl Pts',(-10.3249863758329,-74.3408331090314,
-81.4672909116929));
#31325=CARTESIAN_POINT('Ctrl Pts',(-10.4548672668006,-74.2307923625576,
-81.4883866584888));
#31326=CARTESIAN_POINT('Ctrl Pts',(-10.5796542308205,-74.116914395022,-81.5));
#31327=CARTESIAN_POINT('Ctrl Pts',(-10.6989794855664,-74.,-81.5));
#31328=CARTESIAN_POINT('Ctrl Pts',(-10.7999999953529,-73.1554345313214,
-82.));
#31329=CARTESIAN_POINT('Ctrl Pts',(-11.3926501132988,-72.456338117849,-82.000000001377));
#31330=CARTESIAN_POINT('Ctrl Pts',(-12.2787469320586,-70.9951705629655,
-81.554259559704));
#31331=CARTESIAN_POINT('Ctrl Pts',(-12.6754507792991,-69.4110599090621,
-80.775538373043));
#31332=CARTESIAN_POINT('Ctrl Pts',(-12.7511535426466,-68.7663011286799,
-80.439317485445));
#31333=CARTESIAN_POINT('Ctrl Pts',(-10.9136110332455,-73.2786184794921,
-81.8224303038976));
#31334=CARTESIAN_POINT('Ctrl Pts',(-11.4965284833974,-72.5908737051733,
-81.7864241176491));
#31335=CARTESIAN_POINT('Ctrl Pts',(-12.3544673189724,-71.146729879988,-81.2853611916238));
#31336=CARTESIAN_POINT('Ctrl Pts',(-12.7083706243503,-69.5676980599057,
-80.4850818794619));
#31337=CARTESIAN_POINT('Ctrl Pts',(-12.7661027489825,-68.9230590967111,
-80.1460536890198));
#31338=CARTESIAN_POINT('Ctrl Pts',(-11.0272220711382,-73.4018024276628,
-81.6448606077953));
#31339=CARTESIAN_POINT('Ctrl Pts',(-11.6004068534961,-72.7254092924976,
-81.5728482339212));
#31340=CARTESIAN_POINT('Ctrl Pts',(-12.4301877058861,-71.2982891970106,
-81.0164628235437));
#31341=CARTESIAN_POINT('Ctrl Pts',(-12.7412904694016,-69.7243362107492,
-80.1946253858808));
#31342=CARTESIAN_POINT('Ctrl Pts',(-12.7810519553184,-69.0798170647423,
-79.8527898925946));
#31343=CARTESIAN_POINT('Ctrl Pts',(-11.1408331090309,-73.5249863758335,
-81.467290911693));
#31344=CARTESIAN_POINT('Ctrl Pts',(-11.7042852235948,-72.859944879822,-81.3592723501933));
#31345=CARTESIAN_POINT('Ctrl Pts',(-12.5059080927998,-71.4498485140331,
-80.7475644554636));
#31346=CARTESIAN_POINT('Ctrl Pts',(-12.7742103144529,-69.8809743615928,
-79.9041688922997));
#31347=CARTESIAN_POINT('Ctrl Pts',(-12.7960011616543,-69.2365750327735,
-79.5595260961694));
#31348=CARTESIAN_POINT('Ctrl Pts',(-12.7511535426466,-68.7663011286799,
-80.439317485445));
#31349=CARTESIAN_POINT('Ctrl Pts',(-12.6754507792991,-69.4110599090621,
-80.775538373043));
#31350=CARTESIAN_POINT('Ctrl Pts',(-12.2787469320586,-70.9951705629655,
-81.554259559704));
#31351=CARTESIAN_POINT('Ctrl Pts',(-11.3926501132988,-72.456338117849,-82.000000001377));
#31352=CARTESIAN_POINT('Ctrl Pts',(-10.7999999953529,-73.1554345313214,
-82.));
#31353=CARTESIAN_POINT('',(-11.1408331090314,-73.5249863758329,-81.4672909116929));
#31354=CARTESIAN_POINT('',(-10.7999999970626,-73.1554345327697,-82.));
#31355=CARTESIAN_POINT('Ctrl Pts',(-11.1408331090309,-73.5249863758335,
-81.467290911693));
#31356=CARTESIAN_POINT('Ctrl Pts',(-11.7042852235948,-72.859944879822,-81.3592723501933));
#31357=CARTESIAN_POINT('Ctrl Pts',(-12.5059080927998,-71.4498485140331,
-80.7475644554636));
#31358=CARTESIAN_POINT('Ctrl Pts',(-12.7742103144529,-69.8809743615928,
-79.9041688922997));
#31359=CARTESIAN_POINT('Ctrl Pts',(-12.7960011616543,-69.2365750327735,
-79.5595260961694));
#31360=CARTESIAN_POINT('Ctrl Pts',(-10.4428571428571,-73.5490523794545,
-82.));
#31361=CARTESIAN_POINT('Ctrl Pts',(-10.5665688864269,-73.4227896098978,
-82.));
#31362=CARTESIAN_POINT('Ctrl Pts',(-10.6842569540723,-73.2919662599274,
-82.));
#31363=CARTESIAN_POINT('Ctrl Pts',(-10.7999999953534,-73.1554345313208,
-82.));
#31364=CARTESIAN_POINT('Ctrl Pts',(-10.5619047619048,-73.6656947481584,
-81.8333333333333));
#31365=CARTESIAN_POINT('Ctrl Pts',(-10.6833507226252,-73.5417444835387,
-81.8333333333333));
#31366=CARTESIAN_POINT('Ctrl Pts',(-10.7997687569007,-73.4129332622185,
-81.8294622194963));
#31367=CARTESIAN_POINT('Ctrl Pts',(-10.9136110332461,-73.2786184794915,
-81.8224303038976));
#31368=CARTESIAN_POINT('Ctrl Pts',(-10.6809523809524,-73.7823371168624,
-81.6666666666667));
#31369=CARTESIAN_POINT('Ctrl Pts',(-10.8001325588236,-73.6606993571796,
-81.6666666666667));
#31370=CARTESIAN_POINT('Ctrl Pts',(-10.9152805597292,-73.5339002645096,
-81.6589244389925));
#31371=CARTESIAN_POINT('Ctrl Pts',(-11.0272220711387,-73.4018024276622,
-81.6448606077953));
#31372=CARTESIAN_POINT('Ctrl Pts',(-10.8,-73.8989794855664,-81.5));
#31373=CARTESIAN_POINT('Ctrl Pts',(-10.9169143950219,-73.7796542308205,
-81.5));
#31374=CARTESIAN_POINT('Ctrl Pts',(-11.0307923625576,-73.6548672668006,
-81.4883866584888));
#31375=CARTESIAN_POINT('Ctrl Pts',(-11.1408331090314,-73.5249863758329,
-81.4672909116929));
#31376=CARTESIAN_POINT('Ctrl Pts',(-10.8,-73.8989794855664,-81.5));
#31377=CARTESIAN_POINT('Ctrl Pts',(-10.9169143950219,-73.7796542308205,
-81.5));
#31378=CARTESIAN_POINT('Ctrl Pts',(-11.0307923625576,-73.6548672668006,
-81.4883866584888));
#31379=CARTESIAN_POINT('Ctrl Pts',(-11.1408331090314,-73.5249863758329,
-81.4672909116929));
#31380=CARTESIAN_POINT('Origin',(-10.8,-45.,-80.));
#31381=CARTESIAN_POINT('',(-12.8,-45.,-80.));
#31382=CARTESIAN_POINT('Origin',(-12.8,-37.,-82.));
#31383=CARTESIAN_POINT('',(-12.8,-69.,-82.));
#31384=CARTESIAN_POINT('Origin',(-5.8,-69.,-82.));
#31385=CARTESIAN_POINT('',(-5.8,-76.,-82.));
#31386=CARTESIAN_POINT('Ctrl Pts',(35.9663011250092,-75.9511535430796,-80.4393174835216));
#31387=CARTESIAN_POINT('Ctrl Pts',(35.9605155618968,-75.951832840726,-80.4363004990874));
#31388=CARTESIAN_POINT('Ctrl Pts',(35.9483735247129,-75.9531618864263,-80.4299516020054));
#31389=CARTESIAN_POINT('Ctrl Pts',(35.8779762000419,-75.9616015656904,-80.3933105617495));
#31390=CARTESIAN_POINT('Ctrl Pts',(35.666496759984,-75.9813220332306,-80.282100551774));
#31391=CARTESIAN_POINT('Ctrl Pts',(35.4392833215594,-75.9946945287765,-80.1605539331644));
#31392=CARTESIAN_POINT('Ctrl Pts',(35.227860815934,-76.0000914180091,-80.0472102326352));
#31393=CARTESIAN_POINT('Ctrl Pts',(35.1573138794837,-75.9998884043116,-80.0095380402535));
#31394=CARTESIAN_POINT('Ctrl Pts',(35.1451437858069,-76.,-80.0030795017744));
#31395=CARTESIAN_POINT('Ctrl Pts',(35.1393398282202,-76.,-80.));
#31396=CARTESIAN_POINT('Ctrl Pts',(36.1230590954891,-75.9661027492297,-80.1460536883897));
#31397=CARTESIAN_POINT('Ctrl Pts',(36.11864387275,-75.9664587837152,-80.1437379532279));
#31398=CARTESIAN_POINT('Ctrl Pts',(36.110661351646,-75.9670811329732,-80.139550689276));
#31399=CARTESIAN_POINT('Ctrl Pts',(36.0600402920247,-75.9731109920079,-80.1133005606077));
#31400=CARTESIAN_POINT('Ctrl Pts',(35.8893735775267,-75.9893831955621,-80.0237135233344));
#31401=CARTESIAN_POINT('Ctrl Pts',(35.7265703748804,-75.9981653521971,-79.936367227743));
#31402=CARTESIAN_POINT('Ctrl Pts',(35.55600244748,-76.0010836873959,-79.844739492939));
#31403=CARTESIAN_POINT('Ctrl Pts',(35.5052975502908,-75.9999947733623,-79.8176043516913));
#31404=CARTESIAN_POINT('Ctrl Pts',(35.497312883448,-76.,-79.8133650160679));
#31405=CARTESIAN_POINT('Ctrl Pts',(35.4928932188134,-76.,-79.8110177634954));
#31406=CARTESIAN_POINT('Ctrl Pts',(36.2798170659691,-75.9810519553799,-79.8527898932577));
#31407=CARTESIAN_POINT('Ctrl Pts',(36.2767879876616,-75.9811995800858,-79.8511897097783));
#31408=CARTESIAN_POINT('Ctrl Pts',(36.2691521133615,-75.9816990181399,-79.8471474635063));
#31409=CARTESIAN_POINT('Ctrl Pts',(36.2292067930656,-75.9844912662356,-79.8259370154474));
#31410=CARTESIAN_POINT('Ctrl Pts',(36.1277709673604,-75.9898782465792,-79.7719436231318));
#31411=CARTESIAN_POINT('Ctrl Pts',(35.9983571190163,-75.9966058199617,-79.7030233508242));
#31412=CARTESIAN_POINT('Ctrl Pts',(35.897057117186,-75.9989497585443,-79.6490065320793));
#31413=CARTESIAN_POINT('Ctrl Pts',(35.8571253743265,-75.9998184803151,-79.6277190302889));
#31414=CARTESIAN_POINT('Ctrl Pts',(35.849481981089,-76.,-79.6236505303614));
#31415=CARTESIAN_POINT('Ctrl Pts',(35.8464466094067,-76.,-79.6220355269908));
#31416=CARTESIAN_POINT('Ctrl Pts',(36.436575036449,-75.99600116153,-79.5595260981257));
#31417=CARTESIAN_POINT('Ctrl Pts',(36.4349250886377,-75.9960569557551,-79.5586436598408));
#31418=CARTESIAN_POINT('Ctrl Pts',(36.4314614451549,-75.9961659918624,-79.5567913237265));
#31419=CARTESIAN_POINT('Ctrl Pts',(36.411343857003,-75.9968618284237,-79.5460313716173));
#31420=CARTESIAN_POINT('Ctrl Pts',(36.3508159476629,-75.9984814424111,-79.5136656592577));
#31421=CARTESIAN_POINT('Ctrl Pts',(36.2857765860264,-75.9995667759044,-79.4789019473362));
#31422=CARTESIAN_POINT('Ctrl Pts',(36.225259512466,-76.0000073927787,-79.4465563251417));
#31423=CARTESIAN_POINT('Ctrl Pts',(36.2051143900019,-75.9999908698274,-79.4357876973486));
#31424=CARTESIAN_POINT('Ctrl Pts',(36.20165107873,-76.,-79.4339360446548));
#31425=CARTESIAN_POINT('Ctrl Pts',(36.2,-76.,-79.4330532904862));
#31426=CARTESIAN_POINT('',(35.1393398282202,-76.,-80.));
#31427=CARTESIAN_POINT('',(35.9663011250092,-75.9511535430796,-80.4393174835216));
#31428=CARTESIAN_POINT('Ctrl Pts',(35.1393398282202,-76.,-80.));
#31429=CARTESIAN_POINT('Ctrl Pts',(35.1414419654955,-76.,-80.0011153657435));
#31430=CARTESIAN_POINT('Ctrl Pts',(35.1435480069179,-75.9999991196284,-80.0022328244847));
#31431=CARTESIAN_POINT('Ctrl Pts',(35.1458263157243,-75.9999970367979,-80.003442789511));
#31432=CARTESIAN_POINT('Ctrl Pts',(35.1481625809929,-75.9999949009836,-80.0046835340753));
#31433=CARTESIAN_POINT('Ctrl Pts',(35.1506798636909,-75.9999915030359,-80.0060214842795));
#31434=CARTESIAN_POINT('Ctrl Pts',(35.1535115086618,-75.9999858311707,-80.00752828776));
#31435=CARTESIAN_POINT('Ctrl Pts',(35.1564255209815,-75.9999799943212,-80.0090789213848));
#31436=CARTESIAN_POINT('Ctrl Pts',(35.1596723045489,-75.9999717556759,-80.0108082972711));
#31437=CARTESIAN_POINT('Ctrl Pts',(35.1633488277741,-75.9999592405457,-80.0127685612257));
#31438=CARTESIAN_POINT('Ctrl Pts',(35.1672266124109,-75.9999460403082,-80.0148361345773));
#31439=CARTESIAN_POINT('Ctrl Pts',(35.1715824545328,-75.9999280866369,-80.0171605574455));
#31440=CARTESIAN_POINT('Ctrl Pts',(35.1764781079312,-75.9999022340605,-80.0197750903898));
#31441=CARTESIAN_POINT('Ctrl Pts',(35.1815929833223,-75.999875223834,-80.0225066992533));
#31442=CARTESIAN_POINT('Ctrl Pts',(35.1872968850207,-75.9998395772318,-80.02555487015));
#31443=CARTESIAN_POINT('Ctrl Pts',(35.1936068353733,-75.9997907696175,-80.0289288394651));
#31444=CARTESIAN_POINT('Ctrl Pts',(35.2002790345794,-75.9997391599997,-80.0324965054732));
#31445=CARTESIAN_POINT('Ctrl Pts',(35.2076285905081,-75.9996727937424,-80.0364283067019));
#31446=CARTESIAN_POINT('Ctrl Pts',(35.215620852427,-75.9995857188577,-80.0407056868298));
#31447=CARTESIAN_POINT('Ctrl Pts',(35.2242508253968,-75.9994916961757,-80.0453243636524));
#31448=CARTESIAN_POINT('Ctrl Pts',(35.2336297673748,-75.9993734426237,-80.0503457599988));
#31449=CARTESIAN_POINT('Ctrl Pts',(35.2436568977654,-75.9992237896525,-80.0557156969594));
#31450=CARTESIAN_POINT('Ctrl Pts',(35.2549900980435,-75.9990546438421,-80.0617850875712));
#31451=CARTESIAN_POINT('Ctrl Pts',(35.2671506451442,-75.9988452035161,-80.0682993586211));
#31452=CARTESIAN_POINT('Ctrl Pts',(35.279930567395,-75.9985877512289,-80.0751465277836));
#31453=CARTESIAN_POINT('Ctrl Pts',(35.2990799056129,-75.9982019866815,-80.0854062739348));
#31454=CARTESIAN_POINT('Ctrl Pts',(35.319616549289,-75.9977069524979,-80.0964116738339));
#31455=CARTESIAN_POINT('Ctrl Pts',(35.3407215591454,-75.9970969254858,-80.1077212616672));
#31456=CARTESIAN_POINT('Ctrl Pts',(35.3556136134491,-75.9966664800393,-80.1157014994076));
#31457=CARTESIAN_POINT('Ctrl Pts',(35.3707847308888,-75.996179431309,-80.1238310666215));
#31458=CARTESIAN_POINT('Ctrl Pts',(35.3859667705584,-75.995641541008,-80.1319652977237));
#31459=CARTESIAN_POINT('Ctrl Pts',(35.3988287728834,-75.9951858481991,-80.1388564995401));
#31460=CARTESIAN_POINT('Ctrl Pts',(35.4116980132944,-75.9946938688432,-80.1457507280235));
#31461=CARTESIAN_POINT('Ctrl Pts',(35.4244477602967,-75.9941713808468,-80.1525794999723));
#31462=CARTESIAN_POINT('Ctrl Pts',(35.4361434158036,-75.9936920897979,-80.1588436998998));
#31463=CARTESIAN_POINT('Ctrl Pts',(35.4477381454004,-75.9931872432099,-80.1650526234701));
#31464=CARTESIAN_POINT('Ctrl Pts',(35.4591736956889,-75.9926613511856,-80.1711745877489));
#31465=CARTESIAN_POINT('Ctrl Pts',(35.4699498630682,-75.9921657825131,-80.1769435547067));
#31466=CARTESIAN_POINT('Ctrl Pts',(35.480584408857,-75.9916516129949,-80.1826351629276));
#31467=CARTESIAN_POINT('Ctrl Pts',(35.4910698040367,-75.9911212575979,-80.1882448871593));
#31468=CARTESIAN_POINT('Ctrl Pts',(35.5010892080918,-75.9906144722146,-80.193605304459));
#31469=CARTESIAN_POINT('Ctrl Pts',(35.5109722131649,-75.9900929784058,-80.1988908477128));
#31470=CARTESIAN_POINT('Ctrl Pts',(35.5207544792529,-75.9895564882139,-80.2041200142221));
#31471=CARTESIAN_POINT('Ctrl Pts',(35.5306621203173,-75.9890131220645,-80.209416200645));
#31472=CARTESIAN_POINT('Ctrl Pts',(35.5404657904044,-75.9884544776616,-80.2146542275518));
#31473=CARTESIAN_POINT('Ctrl Pts',(35.5502537086536,-75.9878764060606,-80.2198804089219));
#31474=CARTESIAN_POINT('Ctrl Pts',(35.5596497849624,-75.9873214765304,-80.2248973693938));
#31475=CARTESIAN_POINT('Ctrl Pts',(35.569039357218,-75.9867481787433,-80.229907658822));
#31476=CARTESIAN_POINT('Ctrl Pts',(35.5785104665749,-75.986150798257,-80.2349574569641));
#31477=CARTESIAN_POINT('Ctrl Pts',(35.5885723484862,-75.9855161553992,-80.2403222427213));
#31478=CARTESIAN_POINT('Ctrl Pts',(35.5987262930655,-75.9848542702665,-80.2457316334919));
#31479=CARTESIAN_POINT('Ctrl Pts',(35.6090221995856,-75.984160477439,-80.2512114642467));
#31480=CARTESIAN_POINT('Ctrl Pts',(35.6196563310098,-75.9834438932224,-80.2568713097704));
#31481=CARTESIAN_POINT('Ctrl Pts',(35.6304415318069,-75.9826932206728,-80.2626060938873));
#31482=CARTESIAN_POINT('Ctrl Pts',(35.6413782845434,-75.9819064399385,-80.2684154677553));
#31483=CARTESIAN_POINT('Ctrl Pts',(35.6529860813519,-75.9810713848617,-80.2745812861723));
#31484=CARTESIAN_POINT('Ctrl Pts',(35.6647642745889,-75.9801955856489,-80.2808309446627));
#31485=CARTESIAN_POINT('Ctrl Pts',(35.676658146721,-75.9792810607757,-80.2871349551246));
#31486=CARTESIAN_POINT('Ctrl Pts',(35.6895927548063,-75.9782865132737,-80.2939905782374));
#31487=CARTESIAN_POINT('Ctrl Pts',(35.702663684587,-75.9772460744072,-80.3009102024669));
#31488=CARTESIAN_POINT('Ctrl Pts',(35.7157431200006,-75.9761688075744,-80.3078259962541));
#31489=CARTESIAN_POINT('Ctrl Pts',(35.7310318138807,-75.9749095786924,-80.3159099426023));
#31490=CARTESIAN_POINT('Ctrl Pts',(35.7463312339615,-75.9735998494339,-80.3239881318513));
#31491=CARTESIAN_POINT('Ctrl Pts',(35.7613715111823,-75.972265188833,-80.3319187022711));
#31492=CARTESIAN_POINT('Ctrl Pts',(35.7804794790594,-75.9705695650414,-80.341994120603));
#31493=CARTESIAN_POINT('Ctrl Pts',(35.7991637087092,-75.9688336276876,-80.3518282593546));
#31494=CARTESIAN_POINT('Ctrl Pts',(35.8168183639804,-75.9671305083855,-80.3611060273369));
#31495=CARTESIAN_POINT('Ctrl Pts',(35.829393637445,-75.9659173897695,-80.3677145092204));
#31496=CARTESIAN_POINT('Ctrl Pts',(35.8414447800648,-75.9647215545568,-80.3740398813488));
#31497=CARTESIAN_POINT('Ctrl Pts',(35.8527752050408,-75.9635718404772,-80.3799810880625));
#31498=CARTESIAN_POINT('Ctrl Pts',(35.8629527294715,-75.9625391128293,-80.3853177613651));
#31499=CARTESIAN_POINT('Ctrl Pts',(35.8725480864178,-75.9615437919771,-80.3903441553417));
#31500=CARTESIAN_POINT('Ctrl Pts',(35.8814527903136,-75.9606047204548,-80.3950052279786));
#31501=CARTESIAN_POINT('Ctrl Pts',(35.8897699115574,-75.9597276141749,-80.3993587367197));
#31502=CARTESIAN_POINT('Ctrl Pts',(35.897484103983,-75.9588996965257,-80.4033933465282));
#31503=CARTESIAN_POINT('Ctrl Pts',(35.904545520922,-75.9581323377042,-80.4070844482868));
#31504=CARTESIAN_POINT('Ctrl Pts',(35.9112600151807,-75.9574026787072,-80.4105942086904));
#31505=CARTESIAN_POINT('Ctrl Pts',(35.9173839964454,-75.956727849829,-80.413793238041));
#31506=CARTESIAN_POINT('Ctrl Pts',(35.9229157472091,-75.9561125509301,-80.4166817587725));
#31507=CARTESIAN_POINT('Ctrl Pts',(35.9284930653801,-75.9554921835499,-80.4195940734899));
#31508=CARTESIAN_POINT('Ctrl Pts',(35.9334676603841,-75.9549324406418,-80.4221903895128));
#31509=CARTESIAN_POINT('Ctrl Pts',(35.9378886056851,-75.9544314048567,-80.424497212841));
#31510=CARTESIAN_POINT('Ctrl Pts',(35.9419030613665,-75.9539764374647,-80.4265919322698));
#31511=CARTESIAN_POINT('Ctrl Pts',(35.9454612713508,-75.9535698408206,-80.4284480890796));
#31512=CARTESIAN_POINT('Ctrl Pts',(35.9486430299948,-75.9532043757702,-80.4301077382148));
#31513=CARTESIAN_POINT('Ctrl Pts',(35.9517529694981,-75.9528471600525,-80.431729925497));
#31514=CARTESIAN_POINT('Ctrl Pts',(35.9545030659806,-75.9525292589017,-80.4331642750445));
#31515=CARTESIAN_POINT('Ctrl Pts',(35.9570112127446,-75.9522381265433,-80.4344724355708));
#31516=CARTESIAN_POINT('Ctrl Pts',(35.9594471641416,-75.9519553742397,-80.4357429415505));
#31517=CARTESIAN_POINT('Ctrl Pts',(35.9616547932761,-75.9516978788852,-80.4368943655269));
#31518=CARTESIAN_POINT('Ctrl Pts',(35.9637855481486,-75.9514484584101,-80.4380056097459));
#31519=CARTESIAN_POINT('Ctrl Pts',(35.9646318594599,-75.9513493914681,-80.4384469831598));
#31520=CARTESIAN_POINT('Ctrl Pts',(35.9654665424835,-75.9512515335318,-80.4388822756706));
#31521=CARTESIAN_POINT('Ctrl Pts',(35.9663011250092,-75.9511535430796,-80.4393174835216));
#31522=CARTESIAN_POINT('Ctrl Pts',(36.436575036449,-75.99600116153,-79.5595260981257));
#31523=CARTESIAN_POINT('Ctrl Pts',(36.2798170659691,-75.9810519553799,-79.8527898932577));
#31524=CARTESIAN_POINT('Ctrl Pts',(36.1230590954891,-75.9661027492297,-80.1460536883897));
#31525=CARTESIAN_POINT('Ctrl Pts',(35.9663011250092,-75.9511535430796,-80.4393174835216));
#31526=CARTESIAN_POINT('',(35.6696699141101,-76.,-79.7165266452431));
#31527=CARTESIAN_POINT('Ctrl Pts',(43.196001093997,-69.2365770335277,-79.5595271661901));
#31528=CARTESIAN_POINT('Ctrl Pts',(43.1961126843307,-69.2332771100941,-79.5577622746199));
#31529=CARTESIAN_POINT('Ctrl Pts',(43.1966307615514,-69.2202659648895,-79.5508022076431));
#31530=CARTESIAN_POINT('Ctrl Pts',(43.1985041525164,-69.1506531111129,-79.5135783507796));
#31531=CARTESIAN_POINT('Ctrl Pts',(43.1995836179015,-69.0859374788893,-79.4789878616826));
#31532=CARTESIAN_POINT('Ctrl Pts',(43.2000780175813,-69.0163539017547,-79.4417963142927));
#31533=CARTESIAN_POINT('Ctrl Pts',(43.2,-69.0033021853673,-79.4348188137443));
#31534=CARTESIAN_POINT('Ctrl Pts',(43.2,-69.,-79.4330532904862));
#31535=CARTESIAN_POINT('Ctrl Pts',(43.1810518330435,-69.0798190558569,-79.8527909486787));
#31536=CARTESIAN_POINT('Ctrl Pts',(43.1813470906731,-69.0737608710949,-79.8495905670201));
#31537=CARTESIAN_POINT('Ctrl Pts',(43.1831740472488,-69.0439770045782,-79.8337975102193));
#31538=CARTESIAN_POINT('Ctrl Pts',(43.188912824146,-68.9277181707527,-79.7718563065885));
#31539=CARTESIAN_POINT('Ctrl Pts',(43.1951966216217,-68.7986156255682,-79.7031092616013));
#31540=CARTESIAN_POINT('Ctrl Pts',(43.1992415012141,-68.6823683684193,-79.6411506361618));
#31541=CARTESIAN_POINT('Ctrl Pts',(43.2,-68.6525173807201,-79.6252655486369));
#31542=CARTESIAN_POINT('Ctrl Pts',(43.2,-68.6464466094067,-79.6220355269908));
#31543=CARTESIAN_POINT('Ctrl Pts',(43.1661025720901,-68.9230610781862,-80.1460547311673));
#31544=CARTESIAN_POINT('Ctrl Pts',(43.1668146627161,-68.9142306057276,-80.1414232476533));
#31545=CARTESIAN_POINT('Ctrl Pts',(43.1714769770856,-68.8853775299869,-80.1262741492686));
#31546=CARTESIAN_POINT('Ctrl Pts',(43.1845646124003,-68.6888003693769,-80.0204490165364));
#31547=CARTESIAN_POINT('Ctrl Pts',(43.1958873942081,-68.5271298441114,-79.934679223929));
#31548=CARTESIAN_POINT('Ctrl Pts',(43.1990099699337,-68.3307264381074,-79.8304589746091));
#31549=CARTESIAN_POINT('Ctrl Pts',(43.2,-68.3017325760729,-79.8157122835296));
#31550=CARTESIAN_POINT('Ctrl Pts',(43.2,-68.2928932188134,-79.8110177634954));
#31551=CARTESIAN_POINT('Ctrl Pts',(43.1511533111366,-68.7663031005154,-80.4393185136558));
#31552=CARTESIAN_POINT('Ctrl Pts',(43.1525119129614,-68.754731946507,-80.4332845306422));
#31553=CARTESIAN_POINT('Ctrl Pts',(43.1587889406164,-68.7091438168554,-80.4097047675585));
#31554=CARTESIAN_POINT('Ctrl Pts',(43.1815951370065,-68.4659235447683,-80.2818322537777));
#31555=CARTESIAN_POINT('Ctrl Pts',(43.1948993614971,-68.2398427871283,-80.160865535625));
#31556=CARTESIAN_POINT('Ctrl Pts',(43.2009549676095,-67.9967484366342,-80.0305417453682));
#31557=CARTESIAN_POINT('Ctrl Pts',(43.2,-67.9509477714257,-80.0061590184223));
#31558=CARTESIAN_POINT('Ctrl Pts',(43.2,-67.9393398282202,-80.));
#31559=CARTESIAN_POINT('',(43.1511533111366,-68.7663031005154,-80.4393185136558));
#31560=CARTESIAN_POINT('Ctrl Pts',(43.1511533111366,-68.7663031005154,-80.4393185136558));
#31561=CARTESIAN_POINT('Ctrl Pts',(43.1661025720901,-68.9230610781862,-80.1460547311673));
#31562=CARTESIAN_POINT('Ctrl Pts',(43.1810518330435,-69.0798190558569,-79.8527909486787));
#31563=CARTESIAN_POINT('Ctrl Pts',(43.196001093997,-69.2365770335277,-79.5595271661901));
#31564=CARTESIAN_POINT('Ctrl Pts',(43.1511533111366,-68.7663031005154,-80.4393185136558));
#31565=CARTESIAN_POINT('Ctrl Pts',(43.1513994418684,-68.7642068155316,-80.4382253687564));
#31566=CARTESIAN_POINT('Ctrl Pts',(43.1516451623629,-68.7621066201391,-80.4371299982191));
#31567=CARTESIAN_POINT('Ctrl Pts',(43.1519098993798,-68.7598339313178,-80.4359446578446));
#31568=CARTESIAN_POINT('Ctrl Pts',(43.1521813747516,-68.7575033957165,-80.4347291469851));
#31569=CARTESIAN_POINT('Ctrl Pts',(43.1524728344425,-68.754991600033,-80.4334190935293));
#31570=CARTESIAN_POINT('Ctrl Pts',(43.1527989364355,-68.7521650332621,-80.4319448041782));
#31571=CARTESIAN_POINT('Ctrl Pts',(43.1531345304441,-68.7492561921827,-80.4304276019414));
#31572=CARTESIAN_POINT('Ctrl Pts',(43.1535068018875,-68.7460141346413,-80.4287365400361));
#31573=CARTESIAN_POINT('Ctrl Pts',(43.1539253137781,-68.7423417830772,-80.4268206510669));
#31574=CARTESIAN_POINT('Ctrl Pts',(43.1543667505413,-68.7384682707015,-80.4247998152338));
#31575=CARTESIAN_POINT('Ctrl Pts',(43.1548596340646,-68.7341160525523,-80.4225288569684));
#31576=CARTESIAN_POINT('Ctrl Pts',(43.1554081743586,-68.729223324886,-80.4199748464511));
#31577=CARTESIAN_POINT('Ctrl Pts',(43.1559813015558,-68.7241112933274,-80.4173063590027));
#31578=CARTESIAN_POINT('Ctrl Pts',(43.1566151483999,-68.7184094245538,-80.4143289817675));
#31579=CARTESIAN_POINT('Ctrl Pts',(43.1573073476303,-68.7121007258372,-80.4110327808245));
#31580=CARTESIAN_POINT('Ctrl Pts',(43.1580393345949,-68.7054294020028,-80.4075471136685));
#31581=CARTESIAN_POINT('Ctrl Pts',(43.1588365034245,-68.6980797573121,-80.4037050492237));
#31582=CARTESIAN_POINT('Ctrl Pts',(43.1596890414966,-68.690086577135,-80.3995232917343));
#31583=CARTESIAN_POINT('Ctrl Pts',(43.1606097221028,-68.6814545098864,-80.3950072904599));
#31584=CARTESIAN_POINT('Ctrl Pts',(43.1615948484962,-68.6720723157448,-80.3900953072764));
#31585=CARTESIAN_POINT('Ctrl Pts',(43.1626256551377,-68.6620410817876,-80.3848383268276));
#31586=CARTESIAN_POINT('Ctrl Pts',(43.1637911171991,-68.6506994565633,-80.3788946211662));
#31587=CARTESIAN_POINT('Ctrl Pts',(43.1650147154216,-68.6385288454846,-80.372510219102));
#31588=CARTESIAN_POINT('Ctrl Pts',(43.1662645146486,-68.6257379777259,-80.3657920972819));
#31589=CARTESIAN_POINT('Ctrl Pts',(43.1681310668085,-68.6066350519702,-80.3557587058991));
#31590=CARTESIAN_POINT('Ctrl Pts',(43.1700542679474,-68.5861519923503,-80.3449823921449));
#31591=CARTESIAN_POINT('Ctrl Pts',(43.1719331684166,-68.565102199597,-80.3338855781529));
#31592=CARTESIAN_POINT('Ctrl Pts',(43.1732621227338,-68.5502135913843,-80.3260367542775));
#31593=CARTESIAN_POINT('Ctrl Pts',(43.1745690761519,-68.5350453719404,-80.3180297742375));
#31594=CARTESIAN_POINT('Ctrl Pts',(43.1758280745152,-68.5198657538218,-80.3100055160115));
#31595=CARTESIAN_POINT('Ctrl Pts',(43.1768947566655,-68.5070048731671,-80.3032069900815));
#31596=CARTESIAN_POINT('Ctrl Pts',(43.1779271418599,-68.4941364123874,-80.29639641498));
#31597=CARTESIAN_POINT('Ctrl Pts',(43.1789158885652,-68.4813871493945,-80.2896409949996));
#31598=CARTESIAN_POINT('Ctrl Pts',(43.1798229123759,-68.4696916514037,-80.2834439308359));
#31599=CARTESIAN_POINT('Ctrl Pts',(43.1806932835284,-68.4580968361145,-80.2772934958992));
#31600=CARTESIAN_POINT('Ctrl Pts',(43.181524458385,-68.4466609582864,-80.2712209815302));
#31601=CARTESIAN_POINT('Ctrl Pts',(43.1823077173719,-68.4358843400914,-80.2654985376722));
#31602=CARTESIAN_POINT('Ctrl Pts',(43.1830562233882,-68.4252491329023,-80.2598454426525));
#31603=CARTESIAN_POINT('Ctrl Pts',(43.1837713308511,-68.4147628220254,-80.2542662126462));
#31604=CARTESIAN_POINT('Ctrl Pts',(43.1844546632428,-68.4047424596818,-80.2489348900373));
#31605=CARTESIAN_POINT('Ctrl Pts',(43.1851075444777,-68.3948582667332,-80.2436711326619));
#31606=CARTESIAN_POINT('Ctrl Pts',(43.1857337373957,-68.3850744950793,-80.2384565456612));
#31607=CARTESIAN_POINT('Ctrl Pts',(43.1863647907485,-68.3752147829538,-80.2332014836565));
#31608=CARTESIAN_POINT('Ctrl Pts',(43.1869687712988,-68.3654576384838,-80.22799667205));
#31609=CARTESIAN_POINT('Ctrl Pts',(43.1875516791354,-68.3557161444516,-80.2227965950508));
#31610=CARTESIAN_POINT('Ctrl Pts',(43.1881141226466,-68.3463166480572,-80.2177790787598));
#31611=CARTESIAN_POINT('Ctrl Pts',(43.1886574246308,-68.3369237696628,-80.2127617589513));
#31612=CARTESIAN_POINT('Ctrl Pts',(43.1891861239027,-68.3274492245738,-80.207698253418));
#31613=CARTESIAN_POINT('Ctrl Pts',(43.189747700684,-68.3173854987134,-80.2023198704875));
#31614=CARTESIAN_POINT('Ctrl Pts',(43.1902927448343,-68.3072295951318,-80.1968893513584));
#31615=CARTESIAN_POINT('Ctrl Pts',(43.1908223093172,-68.2969314391131,-80.1913805965219));
#31616=CARTESIAN_POINT('Ctrl Pts',(43.1913689429552,-68.2863013484035,-80.1856942810786));
#31617=CARTESIAN_POINT('Ctrl Pts',(43.1918989882302,-68.2755200646424,-80.1799247984871));
#31618=CARTESIAN_POINT('Ctrl Pts',(43.1924103020824,-68.2645869652587,-80.1740723647106));
#31619=CARTESIAN_POINT('Ctrl Pts',(43.1929529619959,-68.252983612953,-80.1678611478753));
#31620=CARTESIAN_POINT('Ctrl Pts',(43.1934744148126,-68.2412095829377,-80.1615566624412));
#31621=CARTESIAN_POINT('Ctrl Pts',(43.1939700334758,-68.229319364284,-80.1551886129862));
#31622=CARTESIAN_POINT('Ctrl Pts',(43.1945089656157,-68.2163900267524,-80.1482640421924));
#31623=CARTESIAN_POINT('Ctrl Pts',(43.19501719835,-68.203323790513,-80.1412645651496));
#31624=CARTESIAN_POINT('Ctrl Pts',(43.1954885369985,-68.1902480955167,-80.1342590730923));
#31625=CARTESIAN_POINT('Ctrl Pts',(43.1960391678088,-68.174972707951,-80.1260750640363));
#31626=CARTESIAN_POINT('Ctrl Pts',(43.1965391539288,-68.1596853033743,-80.1178833208403));
#31627=CARTESIAN_POINT('Ctrl Pts',(43.1969821282773,-68.1446546577931,-80.1098288638793));
#31628=CARTESIAN_POINT('Ctrl Pts',(43.1975461199478,-68.1255177507933,-80.0995739887334));
#31629=CARTESIAN_POINT('Ctrl Pts',(43.1980169438006,-68.1068025039952,-80.089544602134));
#31630=CARTESIAN_POINT('Ctrl Pts',(43.1983966220753,-68.0891166514876,-80.0800683512888));
#31631=CARTESIAN_POINT('Ctrl Pts',(43.1986667707054,-68.0765328163152,-80.0733258106827));
#31632=CARTESIAN_POINT('Ctrl Pts',(43.1988912194173,-68.064471896412,-80.0668642525555));
#31633=CARTESIAN_POINT('Ctrl Pts',(43.1990759421801,-68.0531305805652,-80.0607896158622));
#31634=CARTESIAN_POINT('Ctrl Pts',(43.1992418556549,-68.0429440876176,-80.0553335255222));
#31635=CARTESIAN_POINT('Ctrl Pts',(43.199375843044,-68.0333387711587,-80.0501899245556));
#31636=CARTESIAN_POINT('Ctrl Pts',(43.1994842520891,-68.0244232494789,-80.0454172395453));
#31637=CARTESIAN_POINT('Ctrl Pts',(43.19958550428,-68.0160963049589,-80.0409596335049));
#31638=CARTESIAN_POINT('Ctrl Pts',(43.19966451597,-68.0083714998843,-80.0368258070954));
#31639=CARTESIAN_POINT('Ctrl Pts',(43.1997270278736,-68.0012988661359,-80.0330426087322));
#31640=CARTESIAN_POINT('Ctrl Pts',(43.1997864675076,-67.9945738307958,-80.0294453430465));
#31641=CARTESIAN_POINT('Ctrl Pts',(43.1998310313963,-67.988438740201,-80.0261652479031));
#31642=CARTESIAN_POINT('Ctrl Pts',(43.1998653972212,-67.9828955516842,-80.0232032971225));
#31643=CARTESIAN_POINT('Ctrl Pts',(43.1999000951797,-67.9772987902027,-80.0202127201308));
#31644=CARTESIAN_POINT('Ctrl Pts',(43.1999244270673,-67.9723061372493,-80.0175468458575));
#31645=CARTESIAN_POINT('Ctrl Pts',(43.1999423966778,-67.9678686119472,-80.0151792611982));
#31646=CARTESIAN_POINT('Ctrl Pts',(43.1999586896024,-67.9638451376985,-80.0130325881632));
#31647=CARTESIAN_POINT('Ctrl Pts',(43.1999697470085,-67.9602777466404,-80.0111309831634));
#31648=CARTESIAN_POINT('Ctrl Pts',(43.1999777607848,-67.957086927538,-80.0094316682685));
#31649=CARTESIAN_POINT('Ctrl Pts',(43.1999855936941,-67.9539681236462,-80.0077707060711));
#31650=CARTESIAN_POINT('Ctrl Pts',(43.1999905148514,-67.9512092797228,-80.0063031091168));
#31651=CARTESIAN_POINT('Ctrl Pts',(43.1999938354518,-67.9486928446362,-80.0049656978208));
#31652=CARTESIAN_POINT('Ctrl Pts',(43.1999970603769,-67.9462489147332,-80.0036668208992));
#31653=CARTESIAN_POINT('Ctrl Pts',(43.1999987706602,-67.9440337265024,-80.0024907890072));
#31654=CARTESIAN_POINT('Ctrl Pts',(43.1999995399948,-67.9418962364246,-80.0013564736068));
#31655=CARTESIAN_POINT('Ctrl Pts',(43.1999998496094,-67.9410360149467,-80.0008999744257));
#31656=CARTESIAN_POINT('Ctrl Pts',(43.2,-67.9401878687046,-80.0004499588664));
#31657=CARTESIAN_POINT('Ctrl Pts',(43.2,-67.9393398282202,-80.));
#31658=CARTESIAN_POINT('Ctrl Pts',(43.1511533111366,-68.7663031005154,-80.4393185136558));
#31659=CARTESIAN_POINT('Ctrl Pts',(43.0502126432029,-69.6260104798524,-80.8876281394629));
#31660=CARTESIAN_POINT('Ctrl Pts',(42.5730796190186,-71.2326776145779,-81.6649032134517));
#31661=CARTESIAN_POINT('Ctrl Pts',(41.6444873881411,-72.631112452033,-82.0000000010328));
#31662=CARTESIAN_POINT('Ctrl Pts',(41.1999999953529,-73.1554345313214,-82.));
#31663=CARTESIAN_POINT('Ctrl Pts',(43.1661025720901,-68.9230610781862,-80.1460547311673));
#31664=CARTESIAN_POINT('Ctrl Pts',(43.0891242241624,-69.7825891654741,-80.5980971278088));
#31665=CARTESIAN_POINT('Ctrl Pts',(42.6545098059633,-71.3823204079613,-81.4026261411462));
#31666=CARTESIAN_POINT('Ctrl Pts',(41.7507989284016,-72.762810125821,-81.7954256760992));
#31667=CARTESIAN_POINT('Ctrl Pts',(41.3136110332455,-73.2786184794921,-81.8224303038976));
#31668=CARTESIAN_POINT('Ctrl Pts',(43.1810518330435,-69.0798190558569,-79.8527909486787));
#31669=CARTESIAN_POINT('Ctrl Pts',(43.1280358051219,-69.9391678510958,-80.3085661161548));
#31670=CARTESIAN_POINT('Ctrl Pts',(42.735939992908,-71.5319632013446,-81.1403490688406));
#31671=CARTESIAN_POINT('Ctrl Pts',(41.8571104686622,-72.894507799609,-81.5908513511656));
#31672=CARTESIAN_POINT('Ctrl Pts',(41.4272220711382,-73.4018024276628,-81.6448606077953));
#31673=CARTESIAN_POINT('Ctrl Pts',(43.196001093997,-69.2365770335277,-79.5595271661901));
#31674=CARTESIAN_POINT('Ctrl Pts',(43.1669473860814,-70.0957465367175,-80.0190351045006));
#31675=CARTESIAN_POINT('Ctrl Pts',(42.8173701798526,-71.6816059947279,-80.8780719965351));
#31676=CARTESIAN_POINT('Ctrl Pts',(41.9634220089227,-73.0262054733971,-81.386277026232));
#31677=CARTESIAN_POINT('Ctrl Pts',(41.5408331090309,-73.5249863758335,-81.467290911693));
#31678=CARTESIAN_POINT('',(41.5408331090314,-73.5249863758329,-81.4672909116929));
#31679=CARTESIAN_POINT('Ctrl Pts',(41.1999999953529,-73.1554345313214,-82.));
#31680=CARTESIAN_POINT('Ctrl Pts',(41.6444873881411,-72.631112452033,-82.0000000010328));
#31681=CARTESIAN_POINT('Ctrl Pts',(42.5730796190186,-71.2326776145779,-81.6649032134517));
#31682=CARTESIAN_POINT('Ctrl Pts',(43.0502126432029,-69.6260104798524,-80.8876281394629));
#31683=CARTESIAN_POINT('Ctrl Pts',(43.1511533111366,-68.7663031005154,-80.4393185136558));
#31684=CARTESIAN_POINT('Origin',(36.2,-69.,-81.75));
#31685=CARTESIAN_POINT('',(40.8428571428571,-73.5490523794545,-82.));
#31686=CARTESIAN_POINT('',(41.0989794855664,-74.,-81.5));
#31687=CARTESIAN_POINT('Ctrl Pts',(41.1999999953534,-73.1554345313208,-82.));
#31688=CARTESIAN_POINT('Ctrl Pts',(41.0842569540723,-73.2919662599274,-82.));
#31689=CARTESIAN_POINT('Ctrl Pts',(40.9665688864269,-73.4227896098978,-82.));
#31690=CARTESIAN_POINT('Ctrl Pts',(40.8428571428571,-73.5490523794545,-82.));
#31691=CARTESIAN_POINT('Ctrl Pts',(41.3136110332461,-73.2786184794915,-81.8224303038976));
#31692=CARTESIAN_POINT('Ctrl Pts',(41.1997687569007,-73.4129332622185,-81.8294622194963));
#31693=CARTESIAN_POINT('Ctrl Pts',(41.0833507226253,-73.5417444835387,-81.8333333333333));
#31694=CARTESIAN_POINT('Ctrl Pts',(40.9619047619048,-73.6656947481584,-81.8333333333333));
#31695=CARTESIAN_POINT('Ctrl Pts',(41.4272220711387,-73.4018024276622,-81.6448606077953));
#31696=CARTESIAN_POINT('Ctrl Pts',(41.3152805597292,-73.5339002645095,-81.6589244389925));
#31697=CARTESIAN_POINT('Ctrl Pts',(41.2001325588236,-73.6606993571796,-81.6666666666667));
#31698=CARTESIAN_POINT('Ctrl Pts',(41.0809523809524,-73.7823371168624,-81.6666666666667));
#31699=CARTESIAN_POINT('Ctrl Pts',(41.5408331090314,-73.5249863758329,-81.4672909116929));
#31700=CARTESIAN_POINT('Ctrl Pts',(41.4307923625576,-73.6548672668006,-81.4883866584888));
#31701=CARTESIAN_POINT('Ctrl Pts',(41.316914395022,-73.7796542308205,-81.5));
#31702=CARTESIAN_POINT('Ctrl Pts',(41.2,-73.8989794855663,-81.5));
#31703=CARTESIAN_POINT('Ctrl Pts',(40.3554345313214,-73.9999999953529,-82.));
#31704=CARTESIAN_POINT('Ctrl Pts',(39.8311122212171,-74.4444875838123,-82.0000000010328));
#31705=CARTESIAN_POINT('Ctrl Pts',(38.4326814201376,-75.3730796207261,-81.6649053966967));
#31706=CARTESIAN_POINT('Ctrl Pts',(36.8259866688679,-75.8502156818532,-80.8876157483302));
#31707=CARTESIAN_POINT('Ctrl Pts',(35.9663011250092,-75.9511535430796,-80.4393174835216));
#31708=CARTESIAN_POINT('Ctrl Pts',(40.4786184794921,-74.1136110332455,-81.8224303038976));
#31709=CARTESIAN_POINT('Ctrl Pts',(39.962809898753,-74.5507991208595,-81.7954256642113));
#31710=CARTESIAN_POINT('Ctrl Pts',(38.5823210678611,-75.454510028044,-81.4026266222993));
#31711=CARTESIAN_POINT('Ctrl Pts',(36.9825801024867,-75.8891261014565,-80.5980924988281));
#31712=CARTESIAN_POINT('Ctrl Pts',(36.1230590954891,-75.9661027492297,-80.1460536883897));
#31713=CARTESIAN_POINT('Ctrl Pts',(40.6018024276628,-74.2272220711382,-81.6448606077953));
#31714=CARTESIAN_POINT('Ctrl Pts',(40.0945075762889,-74.6571106579066,-81.5908513273897));
#31715=CARTESIAN_POINT('Ctrl Pts',(38.7319607155846,-75.5359404353619,-81.140347847902));
#31716=CARTESIAN_POINT('Ctrl Pts',(37.1391735361055,-75.9280365210599,-80.308569249326));
#31717=CARTESIAN_POINT('Ctrl Pts',(36.2798170659691,-75.9810519553799,-79.8527898932577));
#31718=CARTESIAN_POINT('Ctrl Pts',(40.7249863758336,-74.3408331090309,-81.467290911693));
#31719=CARTESIAN_POINT('Ctrl Pts',(40.2262052538249,-74.7634221949538,-81.3862769905682));
#31720=CARTESIAN_POINT('Ctrl Pts',(38.8816003633081,-75.6173708426798,-80.8780690735046));
#31721=CARTESIAN_POINT('Ctrl Pts',(37.2957669697243,-75.9669469406632,-80.0190459998239));
#31722=CARTESIAN_POINT('Ctrl Pts',(36.436575036449,-75.99600116153,-79.5595260981257));
#31723=CARTESIAN_POINT('Ctrl Pts',(35.9663011250092,-75.9511535430796,-80.4393174835216));
#31724=CARTESIAN_POINT('Ctrl Pts',(36.8259866688679,-75.8502156818532,-80.8876157483302));
#31725=CARTESIAN_POINT('Ctrl Pts',(38.4326814201376,-75.3730796207261,-81.6649053966967));
#31726=CARTESIAN_POINT('Ctrl Pts',(39.8311122212171,-74.4444875838123,-82.0000000010328));
#31727=CARTESIAN_POINT('Ctrl Pts',(40.3554345313214,-73.9999999953529,-82.));
#31728=CARTESIAN_POINT('',(40.3554345327697,-73.9999999970625,-82.));
#31729=CARTESIAN_POINT('Ctrl Pts',(40.7490523794545,-73.6428571428571,-82.));
#31730=CARTESIAN_POINT('Ctrl Pts',(40.6227896098978,-73.7665688864269,-82.));
#31731=CARTESIAN_POINT('Ctrl Pts',(40.4919662599274,-73.8842569540723,-82.));
#31732=CARTESIAN_POINT('Ctrl Pts',(40.3554345313208,-73.9999999953534,-82.));
#31733=CARTESIAN_POINT('Ctrl Pts',(40.8656947481584,-73.7619047619048,-81.8333333333333));
#31734=CARTESIAN_POINT('Ctrl Pts',(40.7417444835387,-73.8833507226252,-81.8333333333333));
#31735=CARTESIAN_POINT('Ctrl Pts',(40.6129332622185,-73.9997687569007,-81.8294622194963));
#31736=CARTESIAN_POINT('Ctrl Pts',(40.4786184794915,-74.1136110332461,-81.8224303038976));
#31737=CARTESIAN_POINT('Ctrl Pts',(40.9823371168624,-73.8809523809524,-81.6666666666667));
#31738=CARTESIAN_POINT('Ctrl Pts',(40.8606993571796,-74.0001325588236,-81.6666666666667));
#31739=CARTESIAN_POINT('Ctrl Pts',(40.7339002645096,-74.1152805597292,-81.6589244389925));
#31740=CARTESIAN_POINT('Ctrl Pts',(40.6018024276622,-74.2272220711388,-81.6448606077953));
#31741=CARTESIAN_POINT('Ctrl Pts',(41.0989794855664,-74.,-81.5));
#31742=CARTESIAN_POINT('Ctrl Pts',(40.9796542308205,-74.116914395022,-81.5));
#31743=CARTESIAN_POINT('Ctrl Pts',(40.8548672668006,-74.2307923625576,-81.4883866584888));
#31744=CARTESIAN_POINT('Ctrl Pts',(40.7249863758329,-74.3408331090314,-81.4672909116929));
#31745=CARTESIAN_POINT('Origin',(41.2,-61.,-80.));
#31746=CARTESIAN_POINT('Origin',(4.7,-74.,-80.));
#31747=CARTESIAN_POINT('',(4.7,-76.,-80.));
#31748=CARTESIAN_POINT('Origin',(-5.8,-76.,-82.));
#31749=CARTESIAN_POINT('Origin',(36.2,-69.,-60.));
#31750=CARTESIAN_POINT('',(40.7,-69.,-79.5));
#31751=CARTESIAN_POINT('',(40.7,-69.,-60.));
#31752=CARTESIAN_POINT('Origin',(36.2,-69.,-79.5));
#31753=CARTESIAN_POINT('Origin',(40.7,-37.,-60.));
#31754=CARTESIAN_POINT('',(40.7,-37.,-79.5));
#31755=CARTESIAN_POINT('',(40.7,-37.,-60.));
#31756=CARTESIAN_POINT('',(40.7,-69.,-79.5));
#31757=CARTESIAN_POINT('Origin',(36.2,-37.,-60.));
#31758=CARTESIAN_POINT('',(36.2,-32.5,-79.5));
#31759=CARTESIAN_POINT('',(36.2,-32.5,-60.));
#31760=CARTESIAN_POINT('Origin',(36.2,-37.,-79.5));
#31761=CARTESIAN_POINT('Origin',(-5.8,-32.5,-60.));
#31762=CARTESIAN_POINT('',(36.2,-32.5,-79.5));
#31763=CARTESIAN_POINT('Origin',(15.2,-53.,-79.5));
#32291=UNCERTAINTY_MEASURE_WITH_UNIT(LENGTH_MEASURE(0.01),#32310,
'DISTANCE_ACCURACY_VALUE',
'Maximum model space distance between geometric entities at asserted c
onnectivities');
#32293=UNCERTAINTY_MEASURE_WITH_UNIT(LENGTH_MEASURE(0.01),#32310,
'DISTANCE_ACCURACY_VALUE',
'Maximum model space distance between geometric entities at asserted c
onnectivities');
#32307=(
GEOMETRIC_REPRESENTATION_CONTEXT(3)
GLOBAL_UNCERTAINTY_ASSIGNED_CONTEXT((#32291))
GLOBAL_UNIT_ASSIGNED_CONTEXT((#32310,#32312,#32313))
REPRESENTATION_CONTEXT('','3D')
);
#32309=(
GEOMETRIC_REPRESENTATION_CONTEXT(3)
GLOBAL_UNCERTAINTY_ASSIGNED_CONTEXT((#32293))
GLOBAL_UNIT_ASSIGNED_CONTEXT((#32310,#32312,#32313))
REPRESENTATION_CONTEXT('','3D')
);
#32310=(
LENGTH_UNIT()
NAMED_UNIT(*)
SI_UNIT(.MILLI.,.METRE.)
);
#32312=(
NAMED_UNIT(*)
PLANE_ANGLE_UNIT()
SI_UNIT($,.RADIAN.)
);
#32313=(
NAMED_UNIT(*)
SI_UNIT($,.STERADIAN.)
SOLID_ANGLE_UNIT()
);
#32327=SHAPE_DEFINITION_REPRESENTATION(#32342,#32374);
#32342=PRODUCT_DEFINITION_SHAPE('',$,#32390);
#32374=SHAPE_REPRESENTATION('',(#14802),#32307);
#32376=PRODUCT_DEFINITION_CONTEXT('part definition',#32423,'design');
#32390=PRODUCT_DEFINITION('2026-10-25-00-35-23-176',
'14_Tethered_Dust_Cap',#32405,#32376);
#32405=PRODUCT_DEFINITION_FORMATION('',$,#32438);
#32423=APPLICATION_CONTEXT(
'Core Data for Automotive Mechanical Design Process');
#32424=PRODUCT_CONTEXT('part definition',#32423,'mechanical');
#32438=PRODUCT('2026-10-25-00-35-23-176','14_Tethered_Dust_Cap',$,(#32424));
#32489=COLOUR_RGB('Sky Blue',0.24,0.69,0.87);
#32490=FILL_AREA_STYLE_COLOUR('',#32489);
#32491=FILL_AREA_STYLE('',(#32490));
#32492=SURFACE_STYLE_FILL_AREA(#32491);
#32493=SURFACE_SIDE_STYLE('',(#32492));
#32494=SURFACE_STYLE_USAGE(.BOTH.,#32493);
#32495=PRESENTATION_STYLE_ASSIGNMENT((#32494));
ENDSEC;
END-ISO-10303-21;
